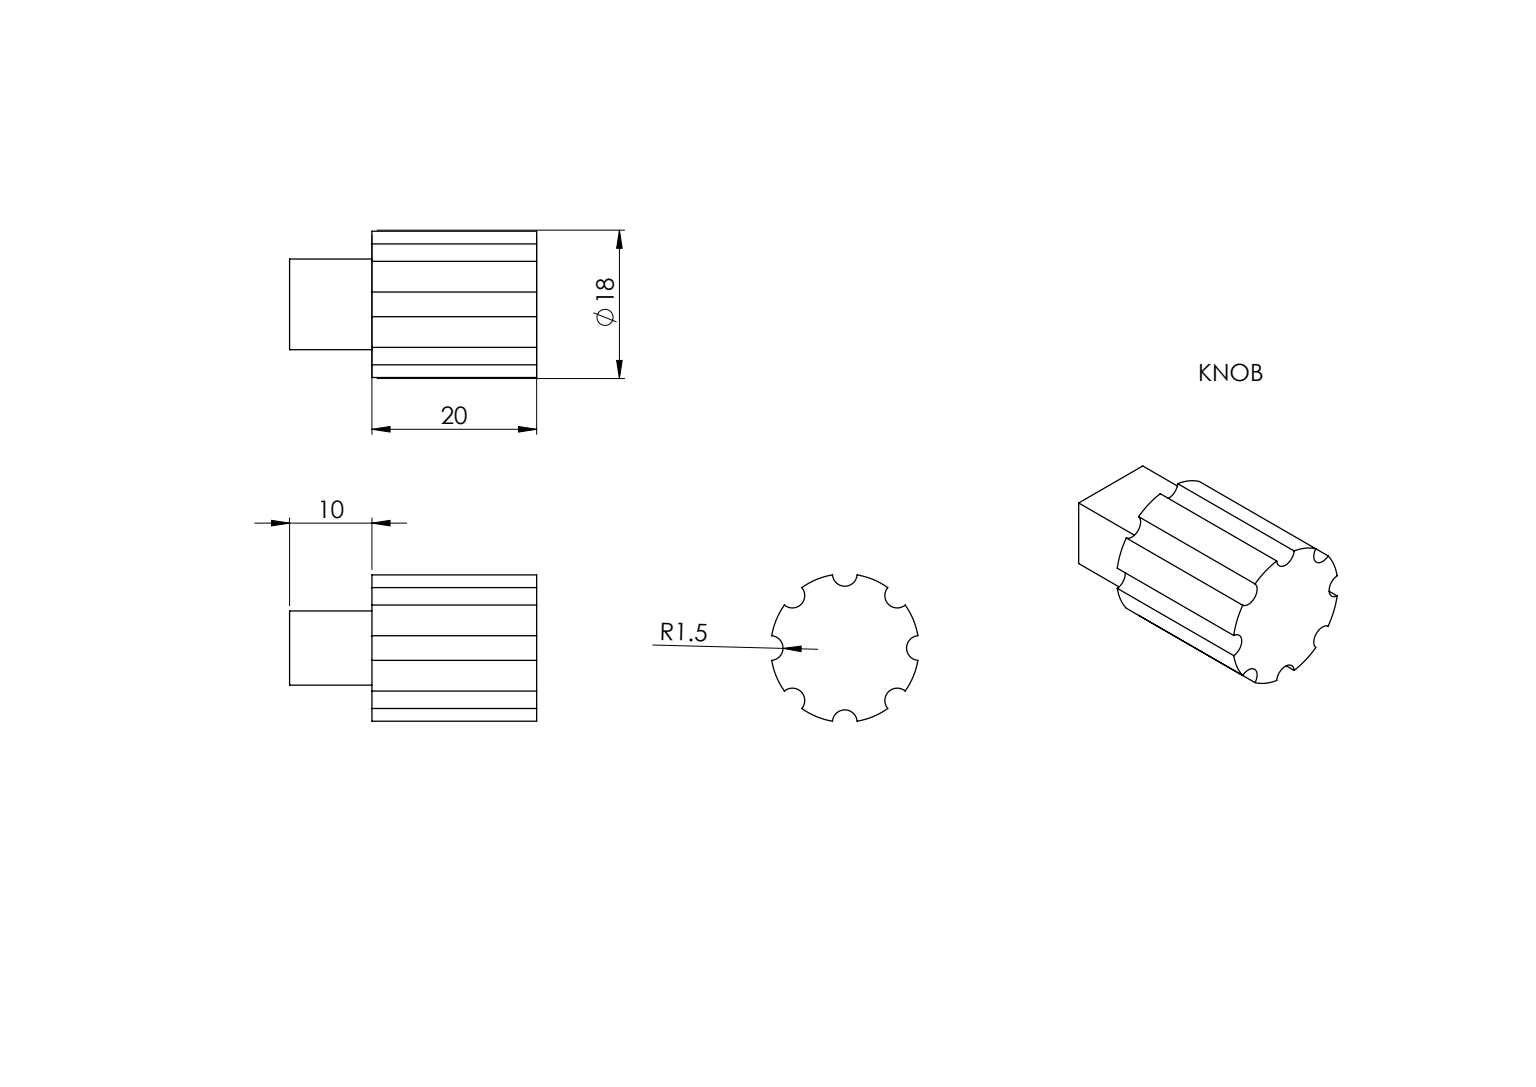
ISO-10303-21;
HEADER;
FILE_DESCRIPTION (('STEP AP214'),
    '1' );
FILE_NAME ('knob.step',
    '2026-10-26T05:42:23',
    ( '' ),
    ( '' ),
    'SwSTEP 2.0',
    'SolidWorks 2026',
    '' );
FILE_SCHEMA (( 'AUTOMOTIVE_DESIGN' ));
ENDSEC;

DATA;
#46=PLANE ( 'NONE',  #66233 ) ;
#122=DIRECTION ( 'NONE',  ( 0.000000000000000000, 0.000000000000000000, -1.000000000000000000 ) ) ;
#188=ORIENTED_EDGE ( 'NONE', *, *, #4935, .T. ) ;
#431=EDGE_CURVE ( 'NONE', #55385, #17600, #60203, .T. ) ;
#446=EDGE_CURVE ( 'NONE', #17600, #24863, #53958, .T. ) ;
#519=EDGE_LOOP ( 'NONE', ( #17956, #34557, #55612, #8707 ) ) ;
#549=DIRECTION ( 'NONE',  ( 0.000000000000000000, 1.000000000000000000, -6.195440985631455317E-17 ) ) ;
#573=EDGE_LOOP ( 'NONE', ( #31473, #72505, #31464, #35325 ) ) ;
#620=AXIS2_PLACEMENT_3D ( 'NONE', #43170, #25435, #32078 ) ;
#671=AXIS2_PLACEMENT_3D ( 'NONE', #60394, #71870, #49704 ) ;
#754=AXIS2_PLACEMENT_3D ( 'NONE', #48020, #47643, #36558 ) ;
#808=DIRECTION ( 'NONE',  ( 0.000000000000000000, 1.000000000000000000, -8.673617379884036705E-17 ) ) ;
#1050=CARTESIAN_POINT ( 'NONE',  ( 65.00000000000000000, 9.000000000000000000, 0.000000000000000000 ) ) ;
#1080=ADVANCED_FACE ( 'NONE', ( #48229 ), #31963, .F. ) ;
#1197=EDGE_CURVE ( 'NONE', #48448, #47360, #14965, .T. ) ;
#1199=DIRECTION ( 'NONE',  ( 0.000000000000000000, 0.000000000000000000, 1.000000000000000000 ) ) ;
#1357=LINE ( 'NONE', #23866, #61936 ) ;
#1404=DIRECTION ( 'NONE',  ( 1.000000000000000000, 0.000000000000000000, 0.000000000000000000 ) ) ;
#1445=DIRECTION ( 'NONE',  ( 1.000000000000000000, 0.000000000000000000, 0.000000000000000000 ) ) ;
#1478=ADVANCED_FACE ( 'NONE', ( #27429 ), #9339, .F. ) ;
#1544=ORIENTED_EDGE ( 'NONE', *, *, #61840, .F. ) ;
#1549=DIRECTION ( 'NONE',  ( 0.000000000000000000, 0.000000000000000000, -1.000000000000000000 ) ) ;
#1681=CARTESIAN_POINT ( 'NONE',  ( 45.00000000000000000, 4.500000000000001776, 5.500000000000000000 ) ) ;
#1739=ORIENTED_EDGE ( 'NONE', *, *, #12260, .F. ) ;
#1799=CARTESIAN_POINT ( 'NONE',  ( 50.00000000000000000, -5.218601775200160553, -7.332543590861066107 ) ) ;
#1839=CARTESIAN_POINT ( 'NONE',  ( 65.00000000000000000, 0.000000000000000000, 0.000000000000000000 ) ) ;
#1840=CARTESIAN_POINT ( 'NONE',  ( 45.00000000000000000, 5.218601775200101045, -7.332543590861111404 ) ) ;
#1886=UNCERTAINTY_MEASURE_WITH_UNIT (LENGTH_MEASURE( 1.000000000000000082E-05 ), #37411, 'distance_accuracy_value', 'NONE');
#1997=VECTOR ( 'NONE', #2916, 1000.000000000000000 ) ;
#2011=DIRECTION ( 'NONE',  ( 0.000000000000000000, 0.000000000000000000, 1.000000000000000000 ) ) ;
#2338=EDGE_CURVE ( 'NONE', #68777, #36937, #65592, .T. ) ;
#2553=CARTESIAN_POINT ( 'NONE',  ( 50.00000000000000000, -5.218601775200058412, 7.332543590861138938 ) ) ;
#2641=VERTEX_POINT ( 'NONE', #50445 ) ;
#2674=EDGE_CURVE ( 'NONE', #33629, #44223, #22352, .T. ) ;
#2860=VECTOR ( 'NONE', #1404, 1000.000000000000000 ) ;
#2916=DIRECTION ( 'NONE',  ( 1.000000000000000000, -0.000000000000000000, -0.000000000000000000 ) ) ;
#3084=DIRECTION ( 'NONE',  ( 0.000000000000000000, 0.000000000000000000, -1.000000000000000000 ) ) ;
#3091=CARTESIAN_POINT ( 'NONE',  ( 45.00000000000000000, 2.500000000000000444, 3.499999999999999112 ) ) ;
#3094=DIRECTION ( 'NONE',  ( 1.000000000000000000, 0.000000000000000000, 0.000000000000000000 ) ) ;
#3140=EDGE_CURVE ( 'NONE', #72600, #46789, #39515, .T. ) ;
#3192=DIRECTION ( 'NONE',  ( 1.000000000000000000, 0.000000000000000000, 0.000000000000000000 ) ) ;
#3258=LINE ( 'NONE', #42776, #39487 ) ;
#3267=ORIENTED_EDGE ( 'NONE', *, *, #14679, .F. ) ;
#3334=EDGE_CURVE ( 'NONE', #68472, #39806, #37194, .T. ) ;
#3337=ORIENTED_EDGE ( 'NONE', *, *, #39334, .T. ) ;
#3340=UNCERTAINTY_MEASURE_WITH_UNIT (LENGTH_MEASURE( 1.000000000000000082E-05 ), #12739, 'distance_accuracy_value', 'NONE');
#3447=EDGE_CURVE ( 'NONE', #60259, #55385, #31156, .T. ) ;
#3560=CYLINDRICAL_SURFACE ( 'NONE', #58366, 9.000000000000000000 ) ;
#3827=ORIENTED_EDGE ( 'NONE', *, *, #69060, .T. ) ;
#3861=( NAMED_UNIT ( * ) PLANE_ANGLE_UNIT ( ) SI_UNIT ( $, .RADIAN. ) );
#3977=ADVANCED_FACE ( 'NONE', ( #20799 ), #51796, .T. ) ;
#4098=VECTOR ( 'NONE', #808, 1000.000000000000000 ) ;
#4198=ORIENTED_EDGE ( 'NONE', *, *, #50924, .F. ) ;
#4229=LINE ( 'NONE', #20454, #24997 ) ;
#4245=CARTESIAN_POINT ( 'NONE',  ( 45.00000000000000000, -8.874999999999998224, -1.494782592887687667 ) ) ;
#4388=CIRCLE ( 'NONE', #39822, 1.500000000000000444 ) ;
#4552=CYLINDRICAL_SURFACE ( 'NONE', #62031, 9.000000000000000000 ) ;
#4729=EDGE_LOOP ( 'NONE', ( #3827, #37731, #11039, #19045 ) ) ;
#4935=EDGE_CURVE ( 'NONE', #51755, #8633, #30167, .T. ) ;
#4977=APPLICATION_CONTEXT ( 'automotive_design' ) ;
#5076=DIRECTION ( 'NONE',  ( 0.000000000000000000, -1.000000000000000000, 8.673617379884035472E-17 ) ) ;
#5100=FACE_OUTER_BOUND ( 'NONE', #43855, .T. ) ;
#5207=DIRECTION ( 'NONE',  ( 0.000000000000000000, 0.000000000000000000, 1.000000000000000000 ) ) ;
#5299=DIRECTION ( 'NONE',  ( 1.000000000000000000, 0.000000000000000000, 0.000000000000000000 ) ) ;
#5322=EDGE_LOOP ( 'NONE', ( #46801, #7370, #39720, #23204 ) ) ;
#5374=CARTESIAN_POINT ( 'NONE',  ( 34.99999999999999289, 4.500000000000000888, -3.500000000000000000 ) ) ;
#5407=DIRECTION ( 'NONE',  ( 1.000000000000000000, 0.000000000000000000, 0.000000000000000000 ) ) ;
#5416=CIRCLE ( 'NONE', #33712, 1.500000000000000444 ) ;
#5432=CARTESIAN_POINT ( 'NONE',  ( 45.00000000000000000, 8.874999999999998224, -1.494782592887687667 ) ) ;
#5621=DIRECTION ( 'NONE',  ( 0.000000000000000000, 0.000000000000000000, -1.000000000000000000 ) ) ;
#5634=ORIENTED_EDGE ( 'NONE', *, *, #39334, .F. ) ;
#5721=FACE_OUTER_BOUND ( 'NONE', #31390, .T. ) ;
#5792=DIRECTION ( 'NONE',  ( 0.000000000000000000, 0.000000000000000000, -1.000000000000000000 ) ) ;
#5818=DIRECTION ( 'NONE',  ( 1.000000000000000000, 0.000000000000000000, 0.000000000000000000 ) ) ;
#6009=ORIENTED_EDGE ( 'NONE', *, *, #59897, .T. ) ;
#6065=LINE ( 'NONE', #50774, #72936 ) ;
#6162=CARTESIAN_POINT ( 'NONE',  ( 20.78732959644809952, -4.500000000000000000, 3.499999999999999556 ) ) ;
#6210=LINE ( 'NONE', #29469, #72836 ) ;
#6340=CARTESIAN_POINT ( 'NONE',  ( 65.00000000000000000, 0.000000000000000000, 0.000000000000000000 ) ) ;
#6410=CARTESIAN_POINT ( 'NONE',  ( 20.78732959644809952, 2.500000000000000000, -3.500000000000000000 ) ) ;
#6440=CARTESIAN_POINT ( 'NONE',  ( 65.00000000000000000, 0.000000000000000000, 0.000000000000000000 ) ) ;
#6514=AXIS2_PLACEMENT_3D ( 'NONE', #1050, #6585, #34643 ) ;
#6563=CARTESIAN_POINT ( 'NONE',  ( 65.00000000000000000, 0.000000000000000000, 0.000000000000000000 ) ) ;
#6585=DIRECTION ( 'NONE',  ( 1.000000000000000000, 0.000000000000000000, 0.000000000000000000 ) ) ;
#6617=FACE_OUTER_BOUND ( 'NONE', #71782, .T. ) ;
#6766=CARTESIAN_POINT ( 'NONE',  ( 34.99999999999999289, 4.500000000000001776, 5.500000000000000000 ) ) ;
#6767=EDGE_CURVE ( 'NONE', #64526, #8633, #16230, .T. ) ;
#6789=DIRECTION ( 'NONE',  ( 1.000000000000000000, 0.000000000000000000, 0.000000000000000000 ) ) ;
#6936=LINE ( 'NONE', #29467, #2860 ) ;
#6938=DIRECTION ( 'NONE',  ( 0.000000000000000000, 0.000000000000000000, -1.000000000000000000 ) ) ;
#7332=CIRCLE ( 'NONE', #48642, 9.000000000000000000 ) ;
#7370=ORIENTED_EDGE ( 'NONE', *, *, #56475, .F. ) ;
#7405=CARTESIAN_POINT ( 'NONE',  ( 65.00000000000000000, 6.363961030679004871, 4.863961030678849440 ) ) ;
#7407=ORIENTED_EDGE ( 'NONE', *, *, #29897, .F. ) ;
#7523=DIRECTION ( 'NONE',  ( 1.000000000000000000, 0.000000000000000000, 0.000000000000000000 ) ) ;
#7603=ORIENTED_EDGE ( 'NONE', *, *, #11775, .F. ) ;
#7713=CIRCLE ( 'NONE', #28956, 9.000000000000000000 ) ;
#7806=ORIENTED_EDGE ( 'NONE', *, *, #32061, .F. ) ;
#7890=DIRECTION ( 'NONE',  ( 0.000000000000000000, 1.000000000000000000, -1.040834085586083941E-14 ) ) ;
#8017=CARTESIAN_POINT ( 'NONE',  ( 34.99999999999999289, -6.363961030678871644, 6.363961030678982667 ) ) ;
#8062=DIRECTION ( 'NONE',  ( 0.000000000000000000, -1.000000000000000000, 8.673617379884035472E-17 ) ) ;
#8100=CARTESIAN_POINT ( 'NONE',  ( 50.00000000000000000, 5.218601775200211179, 7.332543590861028804 ) ) ;
#8189=EDGE_CURVE ( 'NONE', #41205, #2641, #69341, .T. ) ;
#8354=CARTESIAN_POINT ( 'NONE',  ( 45.00000000000000000, 9.000000000000000000, 0.000000000000000000 ) ) ;
#8380=VERTEX_POINT ( 'NONE', #63425 ) ;
#8482=CYLINDRICAL_SURFACE ( 'NONE', #754, 9.000000000000000000 ) ;
#8572=ORIENTED_EDGE ( 'NONE', *, *, #34302, .F. ) ;
#8633=VERTEX_POINT ( 'NONE', #68982 ) ;
#8707=ORIENTED_EDGE ( 'NONE', *, *, #13371, .T. ) ;
#8966=EDGE_CURVE ( 'NONE', #68862, #2641, #49314, .T. ) ;
#9015=EDGE_CURVE ( 'NONE', #24863, #60259, #64072, .T. ) ;
#9059=VECTOR ( 'NONE', #16356, 1000.000000000000000 ) ;
#9220=FACE_OUTER_BOUND ( 'NONE', #11981, .T. ) ;
#9339=PLANE ( 'NONE',  #60749 ) ;
#9386=EDGE_CURVE ( 'NONE', #64526, #47560, #45612, .T. ) ;
#9492=DIRECTION ( 'NONE',  ( 0.000000000000000000, -0.7071067811865487940, -0.7071067811865464625 ) ) ;
#9558=EDGE_CURVE ( 'NONE', #54392, #54059, #19640, .T. ) ;
#9662=PRODUCT_DEFINITION_FORMATION_WITH_SPECIFIED_SOURCE ( 'ANY', '', #23145, .NOT_KNOWN. ) ;
#9854=CARTESIAN_POINT ( 'NONE',  ( 45.00000000000000000, 1.494782592887780703, 8.874999999999982236 ) ) ;
#10069=DIRECTION ( 'NONE',  ( 1.000000000000000000, 0.000000000000000000, -0.000000000000000000 ) ) ;
#10089=DIRECTION ( 'NONE',  ( 1.000000000000000000, 0.000000000000000000, 0.000000000000000000 ) ) ;
#10281=CIRCLE ( 'NONE', #68133, 9.000000000000000000 ) ;
#10315=ORIENTED_EDGE ( 'NONE', *, *, #59108, .T. ) ;
#10378=EDGE_LOOP ( 'NONE', ( #72738, #63812, #49845, #54740 ) ) ;
#10404=ORIENTED_EDGE ( 'NONE', *, *, #2674, .T. ) ;
#10489=DIRECTION ( 'NONE',  ( 0.000000000000000000, 6.195440985631455317E-17, 1.000000000000000000 ) ) ;
#10612=CARTESIAN_POINT ( 'NONE',  ( 20.78732959644809952, 2.500000000000000444, 3.499999999999999112 ) ) ;
#10639=VERTEX_POINT ( 'NONE', #53471 ) ;
#10937=LINE ( 'NONE', #43098, #24203 ) ;
#11039=ORIENTED_EDGE ( 'NONE', *, *, #18886, .F. ) ;
#11110=FACE_OUTER_BOUND ( 'NONE', #11288, .T. ) ;
#11129=ORIENTED_EDGE ( 'NONE', *, *, #67636, .T. ) ;
#11251=VECTOR ( 'NONE', #71053, 1000.000000000000000 ) ;
#11283=DIRECTION ( 'NONE',  ( 0.000000000000000000, 6.195440985631456550E-17, 1.000000000000000000 ) ) ;
#11288=EDGE_LOOP ( 'NONE', ( #69382, #49099, #26689, #56894 ) ) ;
#11325=VECTOR ( 'NONE', #66975, 1000.000000000000000 ) ;
#11376=CARTESIAN_POINT ( 'NONE',  ( 45.00000000000000000, 0.000000000000000000, 0.000000000000000000 ) ) ;
#11404=EDGE_CURVE ( 'NONE', #25148, #8380, #72157, .T. ) ;
#11461=CARTESIAN_POINT ( 'NONE',  ( 34.99999999999999289, -4.500000000000000000, -5.500000000000000000 ) ) ;
#11552=CARTESIAN_POINT ( 'NONE',  ( 65.00000000000000000, 0.000000000000000000, 0.000000000000000000 ) ) ;
#11624=VERTEX_POINT ( 'NONE', #1840 ) ;
#11775=EDGE_CURVE ( 'NONE', #25475, #39806, #52660, .T. ) ;
#11961=PRODUCT_DEFINITION_SHAPE ( 'NONE', 'NONE',  #58930 ) ;
#11981=EDGE_LOOP ( 'NONE', ( #48610, #31142, #50193, #30737 ) ) ;
#11985=CARTESIAN_POINT ( 'NONE',  ( 34.99999999999999289, -4.500000000000000000, 5.500000000000000000 ) ) ;
#12003=ORIENTED_EDGE ( 'NONE', *, *, #3447, .F. ) ;
#12064=CARTESIAN_POINT ( 'NONE',  ( 65.00000000000000000, -5.218601775200160553, -7.332543590861065219 ) ) ;
#12198=VERTEX_POINT ( 'NONE', #26552 ) ;
#12221=ORIENTED_EDGE ( 'NONE', *, *, #29224, .T. ) ;
#12260=EDGE_CURVE ( 'NONE', #8633, #25827, #53155, .T. ) ;
#12356=VECTOR ( 'NONE', #39967, 1000.000000000000000 ) ;
#12400=CIRCLE ( 'NONE', #26595, 1.500000000000000222 ) ;
#12443=AXIS2_PLACEMENT_3D ( 'NONE', #40121, #34556, #57084 ) ;
#12590=ADVANCED_FACE ( 'NONE', ( #58268 ), #18742, .T. ) ;
#12739=( LENGTH_UNIT ( ) NAMED_UNIT ( * ) SI_UNIT ( .MILLI., .METRE. ) );
#12784=DIRECTION ( 'NONE',  ( 1.000000000000000000, -0.000000000000000000, -0.000000000000000000 ) ) ;
#12890=FACE_OUTER_BOUND ( 'NONE', #72920, .T. ) ;
#13193=DIRECTION ( 'NONE',  ( 0.000000000000000000, 0.000000000000000000, -1.000000000000000000 ) ) ;
#13214=EDGE_CURVE ( 'NONE', #12198, #11624, #4388, .T. ) ;
#13314=DIRECTION ( 'NONE',  ( 0.000000000000000000, -1.000000000000000000, 8.673617379884035472E-17 ) ) ;
#13329=CYLINDRICAL_SURFACE ( 'NONE', #49034, 1.500000000000000444 ) ;
#13371=EDGE_CURVE ( 'NONE', #11624, #54715, #37815, .T. ) ;
#13381=ORIENTED_EDGE ( 'NONE', *, *, #37950, .F. ) ;
#13440=EDGE_CURVE ( 'NONE', #15065, #70677, #10281, .T. ) ;
#13450=FILL_AREA_STYLE ('',( #69271 ) ) ;
#13621=DIRECTION ( 'NONE',  ( 1.000000000000000000, 0.000000000000000000, 0.000000000000000000 ) ) ;
#13772=DIRECTION ( 'NONE',  ( 0.000000000000000000, -0.7071067811865437980, 0.7071067811865512365 ) ) ;
#13869=DIRECTION ( 'NONE',  ( 1.000000000000000000, 0.000000000000000000, 0.000000000000000000 ) ) ;
#13928=CARTESIAN_POINT ( 'NONE',  ( 65.00000000000000000, 0.000000000000000000, 0.000000000000000000 ) ) ;
#14163=DIRECTION ( 'NONE',  ( 1.000000000000000000, 0.000000000000000000, 0.000000000000000000 ) ) ;
#14201=EDGE_LOOP ( 'NONE', ( #69016, #43451, #47137, #36436 ) ) ;
#14235=ORIENTED_EDGE ( 'NONE', *, *, #60001, .F. ) ;
#14420=EDGE_CURVE ( 'NONE', #38626, #51755, #37426, .T. ) ;
#14618=DIRECTION ( 'NONE',  ( 1.000000000000000000, 0.000000000000000000, 0.000000000000000000 ) ) ;
#14679=EDGE_CURVE ( 'NONE', #68777, #17600, #6210, .T. ) ;
#14680=FACE_OUTER_BOUND ( 'NONE', #55695, .T. ) ;
#14866=CIRCLE ( 'NONE', #39687, 1.500000000000000444 ) ;
#14965=LINE ( 'NONE', #41589, #26542 ) ;
#14988=DIRECTION ( 'NONE',  ( 1.000000000000000000, 0.000000000000000000, 0.000000000000000000 ) ) ;
#15065=VERTEX_POINT ( 'NONE', #22613 ) ;
#15087=CARTESIAN_POINT ( 'NONE',  ( 34.99999999999999289, 2.500000000000000444, 3.499999999999999112 ) ) ;
#15230=DIRECTION ( 'NONE',  ( 0.000000000000000000, 0.000000000000000000, -1.000000000000000000 ) ) ;
#15392=ORIENTED_EDGE ( 'NONE', *, *, #30954, .F. ) ;
#15478=DIRECTION ( 'NONE',  ( 1.000000000000000000, 0.000000000000000000, 0.000000000000000000 ) ) ;
#15536=EDGE_LOOP ( 'NONE', ( #52738, #18696, #62734, #1739 ) ) ;
#15650=PRODUCT_CONTEXT ( 'NONE', #46934, 'mechanical' ) ;
#15706=ORIENTED_EDGE ( 'NONE', *, *, #3447, .T. ) ;
#15709=DIRECTION ( 'NONE',  ( 1.000000000000000000, 0.000000000000000000, 0.000000000000000000 ) ) ;
#15756=ORIENTED_EDGE ( 'NONE', *, *, #42670, .T. ) ;
#15823=AXIS2_PLACEMENT_3D ( 'NONE', #72302, #56041, #56402 ) ;
#15868=AXIS2_PLACEMENT_3D ( 'NONE', #16774, #6789, #16412 ) ;
#16230=CIRCLE ( 'NONE', #61050, 9.000000000000000000 ) ;
#16270=LINE ( 'NONE', #26644, #26503 ) ;
#16356=DIRECTION ( 'NONE',  ( 1.000000000000000000, 0.000000000000000000, 0.000000000000000000 ) ) ;
#16412=DIRECTION ( 'NONE',  ( 0.000000000000000000, 0.000000000000000000, -1.000000000000000000 ) ) ;
#16425=PLANE ( 'NONE',  #32178 ) ;
#16733=DIRECTION ( 'NONE',  ( 1.000000000000000000, -0.000000000000000000, 0.000000000000000000 ) ) ;
#16774=CARTESIAN_POINT ( 'NONE',  ( 45.00000000000000000, 6.363961030679004871, 6.363961030678849440 ) ) ;
#16796=ORIENTED_EDGE ( 'NONE', *, *, #54938, .F. ) ;
#17052=FACE_OUTER_BOUND ( 'NONE', #573, .T. ) ;
#17374=ORIENTED_EDGE ( 'NONE', *, *, #431, .F. ) ;
#17427=AXIS2_PLACEMENT_3D ( 'NONE', #61543, #5407, #27944 ) ;
#17524=DIRECTION ( 'NONE',  ( 0.000000000000000000, 0.000000000000000000, -1.000000000000000000 ) ) ;
#17526=CARTESIAN_POINT ( 'NONE',  ( 65.00000000000000000, -7.332543590861048344, 5.218601775200187198 ) ) ;
#17531=VERTEX_POINT ( 'NONE', #58303 ) ;
#17582=CARTESIAN_POINT ( 'NONE',  ( 34.99999999999999289, 6.363961030679004871, 6.363961030678849440 ) ) ;
#17600=VERTEX_POINT ( 'NONE', #20240 ) ;
#17778=DIRECTION ( 'NONE',  ( 1.000000000000000000, -0.000000000000000000, -0.000000000000000000 ) ) ;
#17956=ORIENTED_EDGE ( 'NONE', *, *, #25821, .F. ) ;
#17981=DIRECTION ( 'NONE',  ( 1.000000000000000000, 0.000000000000000000, 0.000000000000000000 ) ) ;
#18037=CYLINDRICAL_SURFACE ( 'NONE', #65444, 1.500000000000000444 ) ;
#18058=DIRECTION ( 'NONE',  ( 1.000000000000000000, 0.000000000000000000, 0.000000000000000000 ) ) ;
#18191=DIRECTION ( 'NONE',  ( -1.000000000000000000, 0.000000000000000000, -0.000000000000000000 ) ) ;
#18286=EDGE_CURVE ( 'NONE', #25347, #55385, #33884, .T. ) ;
#18312=CARTESIAN_POINT ( 'NONE',  ( 45.00000000000000000, 0.000000000000000000, 0.000000000000000000 ) ) ;
#18357=FACE_BOUND ( 'NONE', #36376, .T. ) ;
#18431=CARTESIAN_POINT ( 'NONE',  ( 45.00000000000000000, -4.500000000000000000, -5.500000000000000000 ) ) ;
#18589=ORIENTED_EDGE ( 'NONE', *, *, #46820, .F. ) ;
#18593=AXIS2_PLACEMENT_3D ( 'NONE', #6340, #36955, #64296 ) ;
#18633=SURFACE_STYLE_FILL_AREA ( #13450 ) ;
#18696=ORIENTED_EDGE ( 'NONE', *, *, #64237, .T. ) ;
#18742=PLANE ( 'NONE',  #30308 ) ;
#18791=DIRECTION ( 'NONE',  ( 0.000000000000000000, 0.000000000000000000, -1.000000000000000000 ) ) ;
#18850=ORIENTED_EDGE ( 'NONE', *, *, #62575, .F. ) ;
#18886=EDGE_CURVE ( 'NONE', #68472, #48472, #36214, .T. ) ;
#19014=( GEOMETRIC_REPRESENTATION_CONTEXT ( 3 ) GLOBAL_UNCERTAINTY_ASSIGNED_CONTEXT ( ( #57285 ) ) GLOBAL_UNIT_ASSIGNED_CONTEXT ( ( #53357, #41912, #64802 ) ) REPRESENTATION_CONTEXT ( 'NONE', 'WORKASPACE' ) );
#19042=ORIENTED_EDGE ( 'NONE', *, *, #67227, .F. ) ;
#19045=ORIENTED_EDGE ( 'NONE', *, *, #26050, .T. ) ;
#19100=ORIENTED_EDGE ( 'NONE', *, *, #446, .T. ) ;
#19228=VERTEX_POINT ( 'NONE', #23050 ) ;
#19492=PLANE ( 'NONE',  #22949 ) ;
#19508=VECTOR ( 'NONE', #51786, 1000.000000000000000 ) ;
#19512=DIRECTION ( 'NONE',  ( 0.000000000000000000, 0.000000000000000000, -1.000000000000000000 ) ) ;
#19629=ORIENTED_EDGE ( 'NONE', *, *, #44872, .T. ) ;
#19640=CIRCLE ( 'NONE', #63305, 1.499999999999999556 ) ;
#19670=CARTESIAN_POINT ( 'NONE',  ( 45.00000000000000000, 0.000000000000000000, 0.000000000000000000 ) ) ;
#19828=FACE_OUTER_BOUND ( 'NONE', #519, .T. ) ;
#20128=DIRECTION ( 'NONE',  ( 0.000000000000000000, 0.000000000000000000, -1.000000000000000000 ) ) ;
#20153=DIRECTION ( 'NONE',  ( 0.000000000000000000, 0.000000000000000000, -1.000000000000000000 ) ) ;
#20217=DIRECTION ( 'NONE',  ( -0.000000000000000000, 8.673617379884035472E-17, 1.000000000000000000 ) ) ;
#20240=CARTESIAN_POINT ( 'NONE',  ( 45.00000000000000000, -2.499999999999999556, -3.499999999999999556 ) ) ;
#20347=ORIENTED_EDGE ( 'NONE', *, *, #45040, .T. ) ;
#20446=DIRECTION ( 'NONE',  ( 0.000000000000000000, 0.000000000000000000, -1.000000000000000000 ) ) ;
#20454=CARTESIAN_POINT ( 'NONE',  ( 34.99999999999999289, 2.500000000000000000, -3.500000000000000000 ) ) ;
#20492=CARTESIAN_POINT ( 'NONE',  ( 45.00000000000000000, -2.499999999999999556, 3.499999999999999556 ) ) ;
#20568=VECTOR ( 'NONE', #48416, 1000.000000000000000 ) ;
#20587=CARTESIAN_POINT ( 'NONE',  ( 65.00000000000000000, 0.000000000000000000, 0.000000000000000000 ) ) ;
#20611=CYLINDRICAL_SURFACE ( 'NONE', #620, 1.500000000000000444 ) ;
#20614=AXIS2_PLACEMENT_3D ( 'NONE', #11552, #39996, #1199 ) ;
#20666=EDGE_LOOP ( 'NONE', ( #33083, #22259, #69325, #19629, #7407, #33543, #69321, #28131, #50552, #68749, #28455, #3337, #39344, #24424, #24054, #38166, #51564, #1544, #56528 ) ) ;
#20714=CIRCLE ( 'NONE', #62022, 1.500000000000000666 ) ;
#20787=LINE ( 'NONE', #43344, #71482 ) ;
#20799=FACE_OUTER_BOUND ( 'NONE', #45469, .T. ) ;
#20862=AXIS2_PLACEMENT_3D ( 'NONE', #64200, #1445, #52040 ) ;
#20958=FACE_OUTER_BOUND ( 'NONE', #36572, .T. ) ;
#20993=LINE ( 'NONE', #15087, #57263 ) ;
#21022=ORIENTED_EDGE ( 'NONE', *, *, #43507, .F. ) ;
#21111=CARTESIAN_POINT ( 'NONE',  ( 65.00000000000000000, 7.332543590861157590, 5.218601775200033543 ) ) ;
#21170=ORIENTED_EDGE ( 'NONE', *, *, #46759, .T. ) ;
#21308=EDGE_CURVE ( 'NONE', #29028, #64526, #6065, .T. ) ;
#21321=LINE ( 'NONE', #66032, #44378 ) ;
#21425=FACE_OUTER_BOUND ( 'NONE', #25476, .T. ) ;
#21560=CARTESIAN_POINT ( 'NONE',  ( 65.00000000000000000, -6.363961030678871644, 6.363961030678982667 ) ) ;
#21587=EDGE_CURVE ( 'NONE', #12198, #59156, #38709, .T. ) ;
#21698=ORIENTED_EDGE ( 'NONE', *, *, #30772, .T. ) ;
#21774=VECTOR ( 'NONE', #15230, 1000.000000000000000 ) ;
#21839=AXIS2_PLACEMENT_3D ( 'NONE', #8017, #59334, #65253 ) ;
#21857=AXIS2_PLACEMENT_3D ( 'NONE', #28003, #39446, #61967 ) ;
#21974=DIRECTION ( 'NONE',  ( 1.000000000000000000, 0.000000000000000000, 0.000000000000000000 ) ) ;
#21999=MANIFOLD_SOLID_BREP ( 'CirPattern1', #47738 ) ;
#22049=CIRCLE ( 'NONE', #44487, 9.000000000000000000 ) ;
#22243=CARTESIAN_POINT ( 'NONE',  ( 50.00000000000000000, 1.494782592887768269, 8.874999999999984013 ) ) ;
#22259=ORIENTED_EDGE ( 'NONE', *, *, #25821, .T. ) ;
#22351=ORIENTED_EDGE ( 'NONE', *, *, #38259, .T. ) ;
#22352=LINE ( 'NONE', #67078, #66677 ) ;
#22381=ADVANCED_FACE ( 'NONE', ( #17052 ), #39609, .T. ) ;
#22393=CARTESIAN_POINT ( 'NONE',  ( 50.00000000000000000, -8.875000000000000000, 1.494782592887675232 ) ) ;
#22496=FACE_OUTER_BOUND ( 'NONE', #50799, .T. ) ;
#22613=CARTESIAN_POINT ( 'NONE',  ( 65.00000000000000000, 8.874999999999998224, 1.494782592887675232 ) ) ;
#22708=EDGE_CURVE ( 'NONE', #48448, #33629, #29952, .T. ) ;
#22935=ORIENTED_EDGE ( 'NONE', *, *, #46820, .T. ) ;
#22949=AXIS2_PLACEMENT_3D ( 'NONE', #53123, #36862, #8062 ) ;
#23012=VECTOR ( 'NONE', #64511, 1000.000000000000000 ) ;
#23030=ORIENTED_EDGE ( 'NONE', *, *, #13214, .T. ) ;
#23040=AXIS2_PLACEMENT_3D ( 'NONE', #45002, #72342, #34621 ) ;
#23043=CARTESIAN_POINT ( 'NONE',  ( 65.00000000000000000, -6.363961030678960462, -6.363961030678893849 ) ) ;
#23047=CIRCLE ( 'NONE', #671, 1.500000000000000222 ) ;
#23050=CARTESIAN_POINT ( 'NONE',  ( 65.00000000000000000, -1.494782592887706096, -8.874999999999992895 ) ) ;
#23072=CARTESIAN_POINT ( 'NONE',  ( 45.00000000000000000, 0.000000000000000000, 0.000000000000000000 ) ) ;
#23100=CARTESIAN_POINT ( 'NONE',  ( 0.000000000000000000, 0.000000000000000000, 0.000000000000000000 ) ) ;
#23145=PRODUCT ( 'knob', 'knob', '', ( #15650 ) ) ;
#23204=ORIENTED_EDGE ( 'NONE', *, *, #41428, .F. ) ;
#23231=VECTOR ( 'NONE', #5818, 1000.000000000000000 ) ;
#23315=CARTESIAN_POINT ( 'NONE',  ( 45.00000000000000000, 4.500000000000000888, -3.500000000000000000 ) ) ;
#23335=FACE_OUTER_BOUND ( 'NONE', #35526, .T. ) ;
#23612=CARTESIAN_POINT ( 'NONE',  ( 34.99999999999999289, -3.142333204958820020E-14, -9.000000000000000000 ) ) ;
#23694=CARTESIAN_POINT ( 'NONE',  ( 34.99999999999999289, 6.363961030679004871, 4.863961030678849440 ) ) ;
#23746=LINE ( 'NONE', #46294, #28538 ) ;
#23765=AXIS2_PLACEMENT_3D ( 'NONE', #23100, #68190, #46012 ) ;
#23780=CARTESIAN_POINT ( 'NONE',  ( 65.00000000000000000, 1.494782592887643924, -8.875000000000003553 ) ) ;
#23866=CARTESIAN_POINT ( 'NONE',  ( 50.00000000000000000, 8.875000000000000000, -1.494782592887675232 ) ) ;
#24025=PRODUCT_DEFINITION_CONTEXT ( 'detailed design', #4977, 'design' ) ;
#24054=ORIENTED_EDGE ( 'NONE', *, *, #11775, .T. ) ;
#24187=DIRECTION ( 'NONE',  ( 0.000000000000000000, 6.195440985631455317E-17, 1.000000000000000000 ) ) ;
#24203=VECTOR ( 'NONE', #27208, 1000.000000000000000 ) ;
#24424=ORIENTED_EDGE ( 'NONE', *, *, #33157, .F. ) ;
#24452=ORIENTED_EDGE ( 'NONE', *, *, #29897, .T. ) ;
#24480=ORIENTED_EDGE ( 'NONE', *, *, #58454, .T. ) ;
#24739=ORIENTED_EDGE ( 'NONE', *, *, #9015, .F. ) ;
#24799=ORIENTED_EDGE ( 'NONE', *, *, #30402, .T. ) ;
#24863=VERTEX_POINT ( 'NONE', #27180 ) ;
#24882=CARTESIAN_POINT ( 'NONE',  ( 65.00000000000000000, -5.218601775200058412, 7.332543590861138050 ) ) ;
#24918=ORIENTED_EDGE ( 'NONE', *, *, #34570, .T. ) ;
#24944=EDGE_CURVE ( 'NONE', #10639, #56113, #51287, .T. ) ;
#24997=VECTOR ( 'NONE', #10489, 1000.000000000000000 ) ;
#25132=CARTESIAN_POINT ( 'NONE',  ( 34.99999999999999289, 2.500000000000000444, 5.500000000000000000 ) ) ;
#25148=VERTEX_POINT ( 'NONE', #33077 ) ;
#25212=CARTESIAN_POINT ( 'NONE',  ( 34.99999999999999289, -2.499999999999999556, 3.499999999999999556 ) ) ;
#25255=EDGE_CURVE ( 'NONE', #25148, #48448, #55980, .T. ) ;
#25347=VERTEX_POINT ( 'NONE', #64043 ) ;
#25435=DIRECTION ( 'NONE',  ( 1.000000000000000000, -0.000000000000000000, -0.000000000000000000 ) ) ;
#25475=VERTEX_POINT ( 'NONE', #17526 ) ;
#25476=EDGE_LOOP ( 'NONE', ( #56251, #14235, #24452, #25615 ) ) ;
#25507=CARTESIAN_POINT ( 'NONE',  ( 45.00000000000000000, 6.363961030679004871, 4.863961030678849440 ) ) ;
#25615=ORIENTED_EDGE ( 'NONE', *, *, #38259, .F. ) ;
#25619=ORIENTED_EDGE ( 'NONE', *, *, #9386, .F. ) ;
#25657=CARTESIAN_POINT ( 'NONE',  ( 45.00000000000000000, 2.500000000000000000, -3.500000000000000000 ) ) ;
#25821=EDGE_CURVE ( 'NONE', #33507, #54715, #30021, .T. ) ;
#25827=VERTEX_POINT ( 'NONE', #24882 ) ;
#26030=CARTESIAN_POINT ( 'NONE',  ( 34.99999999999999289, 9.426999614876460059E-14, 7.499999999999999112 ) ) ;
#26050=EDGE_CURVE ( 'NONE', #68472, #66931, #16270, .T. ) ;
#26142=CARTESIAN_POINT ( 'NONE',  ( 65.00000000000000000, -3.142333204958820020E-14, -9.000000000000000000 ) ) ;
#26412=CARTESIAN_POINT ( 'NONE',  ( 65.00000000000000000, 6.363961030679004871, 6.363961030678849440 ) ) ;
#26499=VECTOR ( 'NONE', #65390, 1000.000000000000000 ) ;
#26503=VECTOR ( 'NONE', #37711, 1000.000000000000000 ) ;
#26534=CIRCLE ( 'NONE', #45370, 1.500000000000000222 ) ;
#26539=FACE_OUTER_BOUND ( 'NONE', #28983, .T. ) ;
#26542=VECTOR ( 'NONE', #13869, 1000.000000000000000 ) ;
#26552=CARTESIAN_POINT ( 'NONE',  ( 45.00000000000000000, 7.332543590861092753, -5.218601775200125914 ) ) ;
#26595=AXIS2_PLACEMENT_3D ( 'NONE', #21560, #48922, #44114 ) ;
#26602=CIRCLE ( 'NONE', #65506, 9.000000000000000000 ) ;
#26608=CIRCLE ( 'NONE', #43165, 1.500000000000000444 ) ;
#26644=CARTESIAN_POINT ( 'NONE',  ( 50.00000000000000000, -8.875000000000000000, -1.494782592887675232 ) ) ;
#26689=ORIENTED_EDGE ( 'NONE', *, *, #35579, .F. ) ;
#26720=DIRECTION ( 'NONE',  ( 0.000000000000000000, 1.000000000000000000, -6.195440985631456550E-17 ) ) ;
#26881=LINE ( 'NONE', #42405, #72473 ) ;
#26896=VECTOR ( 'NONE', #24187, 1000.000000000000000 ) ;
#27067=( NAMED_UNIT ( * ) SI_UNIT ( $, .STERADIAN. ) SOLID_ANGLE_UNIT ( ) );
#27081=DIRECTION ( 'NONE',  ( -1.000000000000000000, -0.000000000000000000, -0.000000000000000000 ) ) ;
#27152=CARTESIAN_POINT ( 'NONE',  ( 45.00000000000000000, 2.500000000000000444, 3.499999999999999112 ) ) ;
#27180=CARTESIAN_POINT ( 'NONE',  ( 45.00000000000000000, 2.500000000000000000, -3.500000000000000000 ) ) ;
#27208=DIRECTION ( 'NONE',  ( 1.000000000000000000, -0.000000000000000000, -0.000000000000000000 ) ) ;
#27330=ADVANCED_FACE ( 'NONE', ( #21425 ), #27715, .F. ) ;
#27429=FACE_OUTER_BOUND ( 'NONE', #36560, .T. ) ;
#27437=AXIS2_PLACEMENT_3D ( 'NONE', #43454, #48625, #59690 ) ;
#27715=CYLINDRICAL_SURFACE ( 'NONE', #35968, 1.500000000000000444 ) ;
#27818=ORIENTED_EDGE ( 'NONE', *, *, #49856, .F. ) ;
#27821=ADVANCED_FACE ( 'NONE', ( #26539 ), #20611, .F. ) ;
#27870=DIRECTION ( 'NONE',  ( 0.000000000000000000, 0.000000000000000000, -1.000000000000000000 ) ) ;
#27944=DIRECTION ( 'NONE',  ( 0.000000000000000000, 0.000000000000000000, -1.000000000000000000 ) ) ;
#28003=CARTESIAN_POINT ( 'NONE',  ( 45.00000000000000000, 0.000000000000000000, 0.000000000000000000 ) ) ;
#28008=AXIS2_PLACEMENT_3D ( 'NONE', #52725, #69368, #6938 ) ;
#28064=CARTESIAN_POINT ( 'NONE',  ( 34.99999999999999289, -9.000000000000000000, 0.000000000000000000 ) ) ;
#28104=ORIENTED_EDGE ( 'NONE', *, *, #69060, .F. ) ;
#28131=ORIENTED_EDGE ( 'NONE', *, *, #59897, .F. ) ;
#28309=ADVANCED_FACE ( 'NONE', ( #5100, #44990 ), #67528, .F. ) ;
#28331=PLANE ( 'NONE',  #31300 ) ;
#28455=ORIENTED_EDGE ( 'NONE', *, *, #33822, .F. ) ;
#28489=MECHANICAL_DESIGN_GEOMETRIC_PRESENTATION_REPRESENTATION('',(#39139),#63903);
#28538=VECTOR ( 'NONE', #18191, 1000.000000000000000 ) ;
#28694=CARTESIAN_POINT ( 'NONE',  ( 50.00000000000000000, 7.332543590861156702, 5.218601775200032655 ) ) ;
#28773=DIRECTION ( 'NONE',  ( 1.000000000000000000, -0.000000000000000000, -0.000000000000000000 ) ) ;
#28872=ADVANCED_FACE ( 'NONE', ( #36068 ), #3560, .T. ) ;
#28956=AXIS2_PLACEMENT_3D ( 'NONE', #1839, #13621, #18791 ) ;
#28964=AXIS2_PLACEMENT_3D ( 'NONE', #37805, #55175, #71431 ) ;
#28983=EDGE_LOOP ( 'NONE', ( #21022, #62018, #18850, #6009 ) ) ;
#29028=VERTEX_POINT ( 'NONE', #53058 ) ;
#29071=ADVANCED_FACE ( 'NONE', ( #59686 ), #31255, .F. ) ;
#29122=AXIS2_PLACEMENT_3D ( 'NONE', #20587, #43513, #66404 ) ;
#29224=EDGE_CURVE ( 'NONE', #36937, #24863, #56652, .T. ) ;
#29467=CARTESIAN_POINT ( 'NONE',  ( 20.78732959644809952, -4.500000000000000000, -5.500000000000000000 ) ) ;
#29469=CARTESIAN_POINT ( 'NONE',  ( 20.78732959644809952, -2.499999999999999556, -3.499999999999999556 ) ) ;
#29591=LINE ( 'NONE', #34764, #4098 ) ;
#29897=EDGE_CURVE ( 'NONE', #15065, #57451, #64284, .T. ) ;
#29901=ORIENTED_EDGE ( 'NONE', *, *, #37581, .T. ) ;
#29952=LINE ( 'NONE', #25132, #53391 ) ;
#29982=VERTEX_POINT ( 'NONE', #52369 ) ;
#30021=CIRCLE ( 'NONE', #71312, 9.000000000000000000 ) ;
#30104=CARTESIAN_POINT ( 'NONE',  ( 45.00000000000000000, 9.426999614876460059E-14, 7.499999999999999112 ) ) ;
#30167=CIRCLE ( 'NONE', #47847, 1.500000000000000444 ) ;
#30249=AXIS2_PLACEMENT_3D ( 'NONE', #66100, #15478, #65364 ) ;
#30308=AXIS2_PLACEMENT_3D ( 'NONE', #47565, #30932, #53473 ) ;
#30386=CARTESIAN_POINT ( 'NONE',  ( 65.00000000000000000, -7.332543590861121174, -5.218601775200084170 ) ) ;
#30402=EDGE_CURVE ( 'NONE', #71147, #39806, #61916, .T. ) ;
#30465=SURFACE_SIDE_STYLE ('',( #18633 ) ) ;
#30538=CARTESIAN_POINT ( 'NONE',  ( 50.00000000000000000, -7.332543590861121174, -5.218601775200084170 ) ) ;
#30563=CARTESIAN_POINT ( 'NONE',  ( 45.00000000000000000, 0.000000000000000000, 0.000000000000000000 ) ) ;
#30710=ORIENTED_EDGE ( 'NONE', *, *, #57824, .F. ) ;
#30737=ORIENTED_EDGE ( 'NONE', *, *, #56475, .T. ) ;
#30772=EDGE_CURVE ( 'NONE', #17531, #56113, #31332, .T. ) ;
#30874=ORIENTED_EDGE ( 'NONE', *, *, #13440, .F. ) ;
#30883=CARTESIAN_POINT ( 'NONE',  ( 65.00000000000000000, 0.000000000000000000, 0.000000000000000000 ) ) ;
#30886=DIRECTION ( 'NONE',  ( 0.000000000000000000, 0.000000000000000000, 1.000000000000000000 ) ) ;
#30932=DIRECTION ( 'NONE',  ( 1.000000000000000000, 0.000000000000000000, 0.000000000000000000 ) ) ;
#30954=EDGE_CURVE ( 'NONE', #38626, #71147, #26602, .T. ) ;
#30956=DIRECTION ( 'NONE',  ( 0.000000000000000000, 0.000000000000000000, -1.000000000000000000 ) ) ;
#31142=ORIENTED_EDGE ( 'NONE', *, *, #34302, .T. ) ;
#31149=PLANE ( 'NONE',  #61989 ) ;
#31156=LINE ( 'NONE', #3091, #11251 ) ;
#31255=PLANE ( 'NONE',  #34820 ) ;
#31289=AXIS2_PLACEMENT_3D ( 'NONE', #23072, #50800, #17524 ) ;
#31299=ORIENTED_EDGE ( 'NONE', *, *, #44872, .F. ) ;
#31300=AXIS2_PLACEMENT_3D ( 'NONE', #6162, #45328, #67864 ) ;
#31332=CIRCLE ( 'NONE', #28964, 1.500000000000000444 ) ;
#31390=EDGE_LOOP ( 'NONE', ( #54504, #12221, #54418, #45493 ) ) ;
#31464=ORIENTED_EDGE ( 'NONE', *, *, #24944, .F. ) ;
#31473=ORIENTED_EDGE ( 'NONE', *, *, #3140, .T. ) ;
#31534=CARTESIAN_POINT ( 'NONE',  ( 65.00000000000000000, 0.000000000000000000, 0.000000000000000000 ) ) ;
#31569=ORIENTED_EDGE ( 'NONE', *, *, #42670, .F. ) ;
#31692=CYLINDRICAL_SURFACE ( 'NONE', #29122, 9.000000000000000000 ) ;
#31825=CYLINDRICAL_SURFACE ( 'NONE', #46307, 1.500000000000000444 ) ;
#31836=ADVANCED_FACE ( 'NONE', ( #12890 ), #35423, .F. ) ;
#31905=DIRECTION ( 'NONE',  ( 1.000000000000000000, 0.000000000000000000, 0.000000000000000000 ) ) ;
#31963=CYLINDRICAL_SURFACE ( 'NONE', #53687, 1.500000000000000444 ) ;
#31991=CARTESIAN_POINT ( 'NONE',  ( 65.00000000000000000, 0.000000000000000000, 0.000000000000000000 ) ) ;
#32022=EDGE_CURVE ( 'NONE', #68374, #60259, #41697, .T. ) ;
#32052=DIRECTION ( 'NONE',  ( 1.000000000000000000, 0.000000000000000000, 0.000000000000000000 ) ) ;
#32057=CARTESIAN_POINT ( 'NONE',  ( 45.00000000000000000, 1.494782592887656580, -8.875000000000001776 ) ) ;
#32061=EDGE_CURVE ( 'NONE', #54392, #11624, #44332, .T. ) ;
#32078=DIRECTION ( 'NONE',  ( 0.000000000000000000, 0.000000000000000000, -1.000000000000000000 ) ) ;
#32153=EDGE_CURVE ( 'NONE', #2641, #70677, #57843, .T. ) ;
#32177=CARTESIAN_POINT ( 'NONE',  ( 45.00000000000000000, -6.363961030678871644, 6.363961030678982667 ) ) ;
#32178=AXIS2_PLACEMENT_3D ( 'NONE', #68148, #549, #38983 ) ;
#32252=CARTESIAN_POINT ( 'NONE',  ( 45.00000000000000000, -9.000000000000000000, 0.000000000000000000 ) ) ;
#32383=DIRECTION ( 'NONE',  ( -1.000000000000000000, 0.000000000000000000, 0.000000000000000000 ) ) ;
#32950=ORIENTED_EDGE ( 'NONE', *, *, #9558, .F. ) ;
#33077=CARTESIAN_POINT ( 'NONE',  ( 34.99999999999999289, 4.500000000000000888, -5.500000000000000888 ) ) ;
#33083=ORIENTED_EDGE ( 'NONE', *, *, #49669, .F. ) ;
#33157=EDGE_CURVE ( 'NONE', #25475, #40213, #23047, .T. ) ;
#33217=ORIENTED_EDGE ( 'NONE', *, *, #21308, .F. ) ;
#33358=CARTESIAN_POINT ( 'NONE',  ( 20.78732959644809952, 4.500000000000000888, -5.500000000000000888 ) ) ;
#33361=CARTESIAN_POINT ( 'NONE',  ( 45.00000000000000000, 0.000000000000000000, 0.000000000000000000 ) ) ;
#33507=VERTEX_POINT ( 'NONE', #23780 ) ;
#33543=ORIENTED_EDGE ( 'NONE', *, *, #13440, .T. ) ;
#33544=VECTOR ( 'NONE', #57194, 1000.000000000000000 ) ;
#33581=CARTESIAN_POINT ( 'NONE',  ( 34.99999999999999289, 9.426999614876460059E-14, 9.000000000000000000 ) ) ;
#33590=CIRCLE ( 'NONE', #43037, 1.500000000000000888 ) ;
#33629=VERTEX_POINT ( 'NONE', #11985 ) ;
#33639=DIRECTION ( 'NONE',  ( -1.000000000000000000, 0.000000000000000000, 0.000000000000000000 ) ) ;
#33665=VECTOR ( 'NONE', #54515, 1000.000000000000000 ) ;
#33712=AXIS2_PLACEMENT_3D ( 'NONE', #47055, #7523, #7890 ) ;
#33822=EDGE_CURVE ( 'NONE', #29028, #17531, #5416, .T. ) ;
#33884=LINE ( 'NONE', #60868, #23231 ) ;
#33931=DIRECTION ( 'NONE',  ( 1.000000000000000000, 0.000000000000000000, 0.000000000000000000 ) ) ;
#34302=EDGE_CURVE ( 'NONE', #54059, #19228, #20787, .T. ) ;
#34310=CARTESIAN_POINT ( 'NONE',  ( 34.99999999999999289, 2.500000000000000000, -3.500000000000000000 ) ) ;
#34487=ADVANCED_FACE ( 'NONE', ( #55154 ), #4552, .T. ) ;
#34556=DIRECTION ( 'NONE',  ( 1.000000000000000000, 0.000000000000000000, 0.000000000000000000 ) ) ;
#34557=ORIENTED_EDGE ( 'NONE', *, *, #37950, .T. ) ;
#34570=EDGE_CURVE ( 'NONE', #47360, #29982, #39624, .T. ) ;
#34621=DIRECTION ( 'NONE',  ( 0.000000000000000000, 1.000000000000000000, -8.673617379884036705E-17 ) ) ;
#34643=DIRECTION ( 'NONE',  ( 0.000000000000000000, 0.000000000000000000, -1.000000000000000000 ) ) ;
#34764=CARTESIAN_POINT ( 'NONE',  ( 34.99999999999999289, -2.499999999999999556, -5.500000000000000000 ) ) ;
#34786=ORIENTED_EDGE ( 'NONE', *, *, #57824, .T. ) ;
#34820=AXIS2_PLACEMENT_3D ( 'NONE', #53797, #3192, #65603 ) ;
#34877=EDGE_LOOP ( 'NONE', ( #12003, #24739, #44270, #17374 ) ) ;
#35138=ADVANCED_FACE ( 'NONE', ( #67325 ), #66582, .F. ) ;
#35325=ORIENTED_EDGE ( 'NONE', *, *, #62575, .T. ) ;
#35423=CYLINDRICAL_SURFACE ( 'NONE', #66752, 1.499999999999999556 ) ;
#35526=EDGE_LOOP ( 'NONE', ( #67566, #25619, #33217, #67516 ) ) ;
#35579=EDGE_CURVE ( 'NONE', #44223, #25148, #29591, .T. ) ;
#35731=DIRECTION ( 'NONE',  ( 0.000000000000000000, 0.000000000000000000, 1.000000000000000000 ) ) ;
#35732=EDGE_CURVE ( 'NONE', #8380, #47360, #56931, .T. ) ;
#35848=CIRCLE ( 'NONE', #15823, 1.500000000000000888 ) ;
#35968=AXIS2_PLACEMENT_3D ( 'NONE', #44714, #66881, #67250 ) ;
#36043=ORIENTED_EDGE ( 'NONE', *, *, #21308, .T. ) ;
#36068=FACE_OUTER_BOUND ( 'NONE', #54143, .T. ) ;
#36075=LINE ( 'NONE', #30538, #23012 ) ;
#36110=ORIENTED_EDGE ( 'NONE', *, *, #66718, .T. ) ;
#36214=CIRCLE ( 'NONE', #20862, 9.000000000000000000 ) ;
#36376=EDGE_LOOP ( 'NONE', ( #58926, #20347, #37529, #64912 ) ) ;
#36400=DIRECTION ( 'NONE',  ( 1.000000000000000000, 0.000000000000000000, 0.000000000000000000 ) ) ;
#36436=ORIENTED_EDGE ( 'NONE', *, *, #35732, .F. ) ;
#36558=DIRECTION ( 'NONE',  ( 0.000000000000000000, 0.000000000000000000, 1.000000000000000000 ) ) ;
#36560=EDGE_LOOP ( 'NONE', ( #41796, #65819, #19100, #41236 ) ) ;
#36572=EDGE_LOOP ( 'NONE', ( #57851, #67697, #30874, #57160 ) ) ;
#36690=DIRECTION ( 'NONE',  ( 0.000000000000000000, 6.195440985631456550E-17, 1.000000000000000000 ) ) ;
#36814=CARTESIAN_POINT ( 'NONE',  ( 34.99999999999999289, -2.499999999999999556, -3.499999999999999556 ) ) ;
#36823=CARTESIAN_POINT ( 'NONE',  ( 45.00000000000000000, 5.218601775200201409, 7.332543590861037686 ) ) ;
#36830=CARTESIAN_POINT ( 'NONE',  ( 50.00000000000000000, -7.332543590861048344, 5.218601775200186310 ) ) ;
#36862=DIRECTION ( 'NONE',  ( -0.000000000000000000, 8.673617379884035472E-17, 1.000000000000000000 ) ) ;
#36937=VERTEX_POINT ( 'NONE', #34310 ) ;
#36955=DIRECTION ( 'NONE',  ( -1.000000000000000000, -0.000000000000000000, -0.000000000000000000 ) ) ;
#37120=DIRECTION ( 'NONE',  ( 0.000000000000000000, 0.7071067811865388020, -0.7071067811865562325 ) ) ;
#37164=FACE_OUTER_BOUND ( 'NONE', #38980, .T. ) ;
#37194=CIRCLE ( 'NONE', #46627, 1.500000000000000444 ) ;
#37411=( LENGTH_UNIT ( ) NAMED_UNIT ( * ) SI_UNIT ( .MILLI., .METRE. ) );
#37426=CIRCLE ( 'NONE', #28008, 1.500000000000000444 ) ;
#37489=AXIS2_PLACEMENT_3D ( 'NONE', #11376, #17981, #61974 ) ;
#37529=ORIENTED_EDGE ( 'NONE', *, *, #61088, .T. ) ;
#37578=ADVANCED_FACE ( 'NONE', ( #53867 ), #19492, .T. ) ;
#37581=EDGE_CURVE ( 'NONE', #29982, #44755, #3258, .T. ) ;
#37711=DIRECTION ( 'NONE',  ( -1.000000000000000000, 0.000000000000000000, 0.000000000000000000 ) ) ;
#37731=ORIENTED_EDGE ( 'NONE', *, *, #41428, .T. ) ;
#37805=CARTESIAN_POINT ( 'NONE',  ( 65.00000000000000000, 9.426999614876460059E-14, 9.000000000000000000 ) ) ;
#37815=LINE ( 'NONE', #45910, #56317 ) ;
#37950=EDGE_CURVE ( 'NONE', #33507, #54392, #50150, .T. ) ;
#38148=ADVANCED_FACE ( 'NONE', ( #51598 ), #28331, .T. ) ;
#38166=ORIENTED_EDGE ( 'NONE', *, *, #3334, .F. ) ;
#38259=EDGE_CURVE ( 'NONE', #59156, #57451, #1357, .T. ) ;
#38339=VECTOR ( 'NONE', #70525, 1000.000000000000000 ) ;
#38420=CARTESIAN_POINT ( 'NONE',  ( 45.00000000000000000, 0.000000000000000000, 0.000000000000000000 ) ) ;
#38462=CARTESIAN_POINT ( 'NONE',  ( 34.99999999999999289, 0.000000000000000000, 0.000000000000000000 ) ) ;
#38526=CARTESIAN_POINT ( 'NONE',  ( 65.00000000000000000, 0.000000000000000000, 0.000000000000000000 ) ) ;
#38626=VERTEX_POINT ( 'NONE', #53035 ) ;
#38709=CIRCLE ( 'NONE', #54047, 9.000000000000000000 ) ;
#38980=EDGE_LOOP ( 'NONE', ( #58263, #44443, #71366, #3267 ) ) ;
#38983=DIRECTION ( 'NONE',  ( 0.000000000000000000, 6.195440985631455317E-17, 1.000000000000000000 ) ) ;
#39072=ORIENTED_EDGE ( 'NONE', *, *, #3334, .T. ) ;
#39139=STYLED_ITEM ( 'NONE', ( #64437 ), #54116 ) ;
#39334=EDGE_CURVE ( 'NONE', #29028, #25827, #44293, .T. ) ;
#39344=ORIENTED_EDGE ( 'NONE', *, *, #65317, .F. ) ;
#39366=ORIENTED_EDGE ( 'NONE', *, *, #67227, .T. ) ;
#39428=DIRECTION ( 'NONE',  ( 0.000000000000000000, 0.000000000000000000, -1.000000000000000000 ) ) ;
#39446=DIRECTION ( 'NONE',  ( 1.000000000000000000, 0.000000000000000000, 0.000000000000000000 ) ) ;
#39465=VERTEX_POINT ( 'NONE', #56370 ) ;
#39487=VECTOR ( 'NONE', #30956, 1000.000000000000000 ) ;
#39515=CIRCLE ( 'NONE', #31289, 9.000000000000000000 ) ;
#39520=VECTOR ( 'NONE', #51480, 1000.000000000000000 ) ;
#39609=CYLINDRICAL_SURFACE ( 'NONE', #18593, 9.000000000000000000 ) ;
#39624=LINE ( 'NONE', #51061, #11325 ) ;
#39655=DIRECTION ( 'NONE',  ( 0.000000000000000000, 0.000000000000000000, -1.000000000000000000 ) ) ;
#39687=AXIS2_PLACEMENT_3D ( 'NONE', #26142, #66774, #49413 ) ;
#39699=DIRECTION ( 'NONE',  ( -1.000000000000000000, 0.000000000000000000, 0.000000000000000000 ) ) ;
#39720=ORIENTED_EDGE ( 'NONE', *, *, #61840, .T. ) ;
#39728=CARTESIAN_POINT ( 'NONE',  ( 65.00000000000000000, 0.000000000000000000, 0.000000000000000000 ) ) ;
#39806=VERTEX_POINT ( 'NONE', #45652 ) ;
#39822=AXIS2_PLACEMENT_3D ( 'NONE', #55907, #5299, #20446 ) ;
#39967=DIRECTION ( 'NONE',  ( 0.000000000000000000, 6.195440985631456550E-17, 1.000000000000000000 ) ) ;
#39996=DIRECTION ( 'NONE',  ( -1.000000000000000000, -0.000000000000000000, -0.000000000000000000 ) ) ;
#40013=CARTESIAN_POINT ( 'NONE',  ( 65.00000000000000000, 0.000000000000000000, 0.000000000000000000 ) ) ;
#40121=CARTESIAN_POINT ( 'NONE',  ( 45.00000000000000000, -6.363961030678960462, -6.363961030678893849 ) ) ;
#40152=DIRECTION ( 'NONE',  ( 1.000000000000000000, -0.000000000000000000, -0.000000000000000000 ) ) ;
#40213=VERTEX_POINT ( 'NONE', #49493 ) ;
#40354=ORIENTED_EDGE ( 'NONE', *, *, #30402, .F. ) ;
#40447=VERTEX_POINT ( 'NONE', #52030 ) ;
#40518=ORIENTED_EDGE ( 'NONE', *, *, #35579, .T. ) ;
#40533=ORIENTED_EDGE ( 'NONE', *, *, #13214, .F. ) ;
#40783=AXIS2_PLACEMENT_3D ( 'NONE', #18312, #56413, #39428 ) ;
#40876=DIRECTION ( 'NONE',  ( 1.000000000000000000, 0.000000000000000000, 0.000000000000000000 ) ) ;
#41039=STYLED_ITEM('',(#73144),#21999);
#41205=VERTEX_POINT ( 'NONE', #70428 ) ;
#41236=ORIENTED_EDGE ( 'NONE', *, *, #29224, .F. ) ;
#41428=EDGE_CURVE ( 'NONE', #40447, #48472, #36075, .T. ) ;
#41589=CARTESIAN_POINT ( 'NONE',  ( 20.78732959644809952, 4.500000000000001776, 5.500000000000000000 ) ) ;
#41697=LINE ( 'NONE', #64221, #56090 ) ;
#41796=ORIENTED_EDGE ( 'NONE', *, *, #2338, .F. ) ;
#41912=( NAMED_UNIT ( * ) PLANE_ANGLE_UNIT ( ) SI_UNIT ( $, .RADIAN. ) );
#42308=LINE ( 'NONE', #70381, #64216 ) ;
#42405=CARTESIAN_POINT ( 'NONE',  ( 45.00000000000000000, -2.499999999999999556, -5.500000000000000000 ) ) ;
#42570=EDGE_LOOP ( 'NONE', ( #68240, #42938, #18589, #55019 ) ) ;
#42670=EDGE_CURVE ( 'NONE', #66931, #71147, #26608, .T. ) ;
#42699=CARTESIAN_POINT ( 'NONE',  ( 34.99999999999999289, -2.499999999999999556, -3.499999999999999556 ) ) ;
#42776=CARTESIAN_POINT ( 'NONE',  ( 45.00000000000000000, -4.500000000000000000, 3.499999999999999556 ) ) ;
#42909=ADVANCED_FACE ( 'NONE', ( #54785 ), #31149, .T. ) ;
#42923=ORIENTED_EDGE ( 'NONE', *, *, #26050, .F. ) ;
#42938=ORIENTED_EDGE ( 'NONE', *, *, #14420, .F. ) ;
#43005=VECTOR ( 'NONE', #11283, 1000.000000000000000 ) ;
#43037=AXIS2_PLACEMENT_3D ( 'NONE', #26412, #36400, #37120 ) ;
#43049=CARTESIAN_POINT ( 'NONE',  ( 34.99999999999999289, 6.363961030678916053, -6.363961030678939146 ) ) ;
#43098=CARTESIAN_POINT ( 'NONE',  ( 34.99999999999999289, -6.363961030678871644, 4.863961030678981778 ) ) ;
#43165=AXIS2_PLACEMENT_3D ( 'NONE', #32252, #10089, #3084 ) ;
#43170=CARTESIAN_POINT ( 'NONE',  ( 34.99999999999999289, 6.363961030679004871, 6.363961030678849440 ) ) ;
#43328=DIRECTION ( 'NONE',  ( 0.000000000000000000, 1.000000000000000000, -8.673617379884036705E-17 ) ) ;
#43344=CARTESIAN_POINT ( 'NONE',  ( 50.00000000000000000, -1.494782592887706318, -8.874999999999994671 ) ) ;
#43451=ORIENTED_EDGE ( 'NONE', *, *, #25255, .T. ) ;
#43454=CARTESIAN_POINT ( 'NONE',  ( 20.78732959644809952, -2.499999999999999556, 3.499999999999999556 ) ) ;
#43507=EDGE_CURVE ( 'NONE', #68862, #51352, #63944, .T. ) ;
#43513=DIRECTION ( 'NONE',  ( -1.000000000000000000, -0.000000000000000000, -0.000000000000000000 ) ) ;
#43521=ADVANCED_FACE ( 'NONE', ( #23335 ), #13329, .F. ) ;
#43818=CARTESIAN_POINT ( 'NONE',  ( 45.00000000000000000, -8.874999999999998224, 1.494782592887687667 ) ) ;
#43845=DIRECTION ( 'NONE',  ( 1.000000000000000000, 0.000000000000000000, 0.000000000000000000 ) ) ;
#43855=EDGE_LOOP ( 'NONE', ( #7806, #71888, #16796, #48163, #28104, #15756, #15392, #62455, #188, #61857, #66700, #39366, #53451, #69955, #46717, #68886, #51923, #50278, #23030 ) ) ;
#44057=CARTESIAN_POINT ( 'NONE',  ( 20.78732959644809952, -2.499999999999999556, -3.499999999999999556 ) ) ;
#44114=DIRECTION ( 'NONE',  ( 0.000000000000000000, 0.7071067811865535679, 0.7071067811865414665 ) ) ;
#44158=AXIS2_PLACEMENT_3D ( 'NONE', #33581, #61654, #66480 ) ;
#44223=VERTEX_POINT ( 'NONE', #11461 ) ;
#44238=VECTOR ( 'NONE', #61945, 1000.000000000000000 ) ;
#44270=ORIENTED_EDGE ( 'NONE', *, *, #446, .F. ) ;
#44293=CIRCLE ( 'NONE', #54867, 9.000000000000000000 ) ;
#44325=CIRCLE ( 'NONE', #12443, 1.500000000000000444 ) ;
#44332=CIRCLE ( 'NONE', #40783, 9.000000000000000000 ) ;
#44343=DIRECTION ( 'NONE',  ( 1.000000000000000000, 0.000000000000000000, 0.000000000000000000 ) ) ;
#44378=VECTOR ( 'NONE', #32052, 1000.000000000000000 ) ;
#44429=VECTOR ( 'NONE', #61760, 1000.000000000000000 ) ;
#44443=ORIENTED_EDGE ( 'NONE', *, *, #18286, .T. ) ;
#44487=AXIS2_PLACEMENT_3D ( 'NONE', #70022, #40876, #46774 ) ;
#44620=CARTESIAN_POINT ( 'NONE',  ( 50.00000000000000000, 1.494782592887643924, -8.875000000000003553 ) ) ;
#44714=CARTESIAN_POINT ( 'NONE',  ( 34.99999999999999289, 9.000000000000000000, 0.000000000000000000 ) ) ;
#44755=VERTEX_POINT ( 'NONE', #18431 ) ;
#44872=EDGE_CURVE ( 'NONE', #71649, #57451, #7713, .T. ) ;
#44904=DIRECTION ( 'NONE',  ( 0.000000000000000000, 0.000000000000000000, -1.000000000000000000 ) ) ;
#44990=FACE_BOUND ( 'NONE', #68012, .T. ) ;
#45002=CARTESIAN_POINT ( 'NONE',  ( 20.78732959644809952, -2.499999999999999556, -5.500000000000000000 ) ) ;
#45040=EDGE_CURVE ( 'NONE', #68374, #25347, #20993, .T. ) ;
#45046=CYLINDRICAL_SURFACE ( 'NONE', #44158, 1.500000000000000444 ) ;
#45111=CIRCLE ( 'NONE', #66300, 1.500000000000000444 ) ;
#45144=CARTESIAN_POINT ( 'NONE',  ( 34.99999999999999289, -6.363961030678960462, -6.363961030678893849 ) ) ;
#45328=DIRECTION ( 'NONE',  ( 0.000000000000000000, -1.000000000000000000, 0.000000000000000000 ) ) ;
#45370=AXIS2_PLACEMENT_3D ( 'NONE', #23043, #58828, #13772 ) ;
#45469=EDGE_LOOP ( 'NONE', ( #54998, #24799, #7603, #22935 ) ) ;
#45493=ORIENTED_EDGE ( 'NONE', *, *, #32022, .F. ) ;
#45503=ADVANCED_FACE ( 'NONE', ( #45728 ), #67539, .T. ) ;
#45548=AXIS2_PLACEMENT_3D ( 'NONE', #39728, #15709, #55615 ) ;
#45612=CIRCLE ( 'NONE', #30249, 1.500000000000000444 ) ;
#45638=ADVANCED_FACE ( 'NONE', ( #62706 ), #57152, .T. ) ;
#45652=CARTESIAN_POINT ( 'NONE',  ( 65.00000000000000000, -8.874999999999998224, 1.494782592887675232 ) ) ;
#45728=FACE_OUTER_BOUND ( 'NONE', #60690, .T. ) ;
#45910=CARTESIAN_POINT ( 'NONE',  ( 50.00000000000000000, 5.218601775200110815, -7.332543590861103411 ) ) ;
#46002=ADVANCED_FACE ( 'NONE', ( #19828 ), #57539, .T. ) ;
#46012=DIRECTION ( 'NONE',  ( 1.000000000000000000, 0.000000000000000000, 0.000000000000000000 ) ) ;
#46096=ORIENTED_EDGE ( 'NONE', *, *, #37581, .F. ) ;
#46128=LINE ( 'NONE', #1799, #33544 ) ;
#46259=ORIENTED_EDGE ( 'NONE', *, *, #18286, .F. ) ;
#46294=CARTESIAN_POINT ( 'NONE',  ( 50.00000000000000000, 7.332543590861084759, -5.218601775200136572 ) ) ;
#46307=AXIS2_PLACEMENT_3D ( 'NONE', #48819, #54724, #48088 ) ;
#46370=CARTESIAN_POINT ( 'NONE',  ( 45.00000000000000000, -1.494782592887594852, 8.875000000000012434 ) ) ;
#46605=CARTESIAN_POINT ( 'NONE',  ( 34.99999999999999289, 9.426999614876460059E-14, 9.000000000000000000 ) ) ;
#46627=AXIS2_PLACEMENT_3D ( 'NONE', #65137, #14163, #2011 ) ;
#46717=ORIENTED_EDGE ( 'NONE', *, *, #8966, .T. ) ;
#46759=EDGE_CURVE ( 'NONE', #71649, #54715, #20714, .T. ) ;
#46774=DIRECTION ( 'NONE',  ( 0.000000000000000000, 0.000000000000000000, -1.000000000000000000 ) ) ;
#46789=VERTEX_POINT ( 'NONE', #9854 ) ;
#46801=ORIENTED_EDGE ( 'NONE', *, *, #47241, .F. ) ;
#46820=EDGE_CURVE ( 'NONE', #25475, #38626, #64902, .T. ) ;
#46934=APPLICATION_CONTEXT ( 'automotive_design' ) ;
#47055=CARTESIAN_POINT ( 'NONE',  ( 65.00000000000000000, 9.426999614876460059E-14, 9.000000000000000000 ) ) ;
#47137=ORIENTED_EDGE ( 'NONE', *, *, #1197, .T. ) ;
#47241=EDGE_CURVE ( 'NONE', #39465, #40447, #44325, .T. ) ;
#47282=CARTESIAN_POINT ( 'NONE',  ( 45.00000000000000000, -6.363961030678871644, 4.863961030678981778 ) ) ;
#47360=VERTEX_POINT ( 'NONE', #1681 ) ;
#47404=VECTOR ( 'NONE', #69998, 1000.000000000000000 ) ;
#47560=VERTEX_POINT ( 'NONE', #30104 ) ;
#47565=CARTESIAN_POINT ( 'NONE',  ( 65.00000000000000000, 0.000000000000000000, 0.000000000000000000 ) ) ;
#47643=DIRECTION ( 'NONE',  ( -1.000000000000000000, -0.000000000000000000, -0.000000000000000000 ) ) ;
#47738=CLOSED_SHELL ( 'NONE', ( #63892, #56255, #58996, #51871, #45638, #3977, #34487, #22381, #54331, #46002, #37578, #42909, #45503, #38148, #50000, #70271, #1478, #70933, #72125, #12590, #28872, #28309, #29071, #27330, #1080, #27821, #43521, #71684, #61479, #35138, #31836 ) ) ;
#47842=AXIS2_PLACEMENT_3D ( 'NONE', #13928, #69003, #35731 ) ;
#47847=AXIS2_PLACEMENT_3D ( 'NONE', #32177, #66522, #49179 ) ;
#47892=DIRECTION ( 'NONE',  ( -1.000000000000000000, -0.000000000000000000, -0.000000000000000000 ) ) ;
#47949=DIRECTION ( 'NONE',  ( 0.000000000000000000, 1.000000000000000000, -8.673617379884036705E-17 ) ) ;
#48020=CARTESIAN_POINT ( 'NONE',  ( 65.00000000000000000, 0.000000000000000000, 0.000000000000000000 ) ) ;
#48088=DIRECTION ( 'NONE',  ( 0.000000000000000000, 0.000000000000000000, -1.000000000000000000 ) ) ;
#48163=ORIENTED_EDGE ( 'NONE', *, *, #47241, .T. ) ;
#48229=FACE_OUTER_BOUND ( 'NONE', #55691, .T. ) ;
#48416=DIRECTION ( 'NONE',  ( 0.000000000000000000, 1.000000000000000000, -8.673617379884036705E-17 ) ) ;
#48448=VERTEX_POINT ( 'NONE', #6766 ) ;
#48472=VERTEX_POINT ( 'NONE', #30386 ) ;
#48610=ORIENTED_EDGE ( 'NONE', *, *, #54938, .T. ) ;
#48625=DIRECTION ( 'NONE',  ( 0.000000000000000000, -1.000000000000000000, 0.000000000000000000 ) ) ;
#48642=AXIS2_PLACEMENT_3D ( 'NONE', #30883, #14618, #20153 ) ;
#48764=EDGE_LOOP ( 'NONE', ( #27818, #10404, #34786, #46096 ) ) ;
#48819=CARTESIAN_POINT ( 'NONE',  ( 34.99999999999999289, -6.363961030678871644, 6.363961030678982667 ) ) ;
#48922=DIRECTION ( 'NONE',  ( 1.000000000000000000, 0.000000000000000000, 0.000000000000000000 ) ) ;
#48977=ORIENTED_EDGE ( 'NONE', *, *, #32022, .T. ) ;
#49034=AXIS2_PLACEMENT_3D ( 'NONE', #46605, #17778, #1549 ) ;
#49053=PLANE ( 'NONE',  #60849 ) ;
#49099=ORIENTED_EDGE ( 'NONE', *, *, #25255, .F. ) ;
#49179=DIRECTION ( 'NONE',  ( 0.000000000000000000, 0.000000000000000000, -1.000000000000000000 ) ) ;
#49235=DIRECTION ( 'NONE',  ( 0.000000000000000000, -8.673617379884036705E-17, -1.000000000000000000 ) ) ;
#49314=CIRCLE ( 'NONE', #17427, 1.500000000000000444 ) ;
#49413=DIRECTION ( 'NONE',  ( 0.000000000000000000, -1.000000000000000000, 3.469446951953613006E-15 ) ) ;
#49493=CARTESIAN_POINT ( 'NONE',  ( 65.00000000000000000, -6.363961030678871644, 4.863961030678981778 ) ) ;
#49496=CARTESIAN_POINT ( 'NONE',  ( 65.00000000000000000, 1.494782592887768269, 8.874999999999982236 ) ) ;
#49612=DIRECTION ( 'NONE',  ( 0.000000000000000000, 0.000000000000000000, 1.000000000000000000 ) ) ;
#49669=EDGE_CURVE ( 'NONE', #33507, #19228, #14866, .T. ) ;
#49704=DIRECTION ( 'NONE',  ( 0.000000000000000000, 0.7071067811865535679, 0.7071067811865414665 ) ) ;
#49711=ORIENTED_EDGE ( 'NONE', *, *, #58454, .F. ) ;
#49752=CARTESIAN_POINT ( 'NONE',  ( 65.00000000000000000, 6.363961030678916053, -6.363961030678939146 ) ) ;
#49778=DIRECTION ( 'NONE',  ( 1.000000000000000000, -0.000000000000000000, -0.000000000000000000 ) ) ;
#49845=ORIENTED_EDGE ( 'NONE', *, *, #49856, .T. ) ;
#49856=EDGE_CURVE ( 'NONE', #33629, #29982, #21321, .T. ) ;
#49871=CARTESIAN_POINT ( 'NONE',  ( 45.00000000000000000, -2.499999999999999556, 3.499999999999999556 ) ) ;
#50000=ADVANCED_FACE ( 'NONE', ( #14680 ), #49053, .F. ) ;
#50084=ORIENTED_EDGE ( 'NONE', *, *, #45040, .F. ) ;
#50150=LINE ( 'NONE', #44620, #44238 ) ;
#50183=DIRECTION ( 'NONE',  ( -1.000000000000000000, -0.000000000000000000, -0.000000000000000000 ) ) ;
#50193=ORIENTED_EDGE ( 'NONE', *, *, #68511, .F. ) ;
#50278=ORIENTED_EDGE ( 'NONE', *, *, #21587, .F. ) ;
#50363=DIRECTION ( 'NONE',  ( 1.000000000000000000, 0.000000000000000000, 0.000000000000000000 ) ) ;
#50445=CARTESIAN_POINT ( 'NONE',  ( 45.00000000000000000, 7.332543590861163807, 5.218601775200022885 ) ) ;
#50552=ORIENTED_EDGE ( 'NONE', *, *, #24944, .T. ) ;
#50774=CARTESIAN_POINT ( 'NONE',  ( 50.00000000000000000, -1.494782592887582195, 8.875000000000014211 ) ) ;
#50799=EDGE_LOOP ( 'NONE', ( #19042, #36110, #21698, #4198 ) ) ;
#50800=DIRECTION ( 'NONE',  ( 1.000000000000000000, 0.000000000000000000, 0.000000000000000000 ) ) ;
#50924=EDGE_CURVE ( 'NONE', #46789, #56113, #67681, .T. ) ;
#51061=CARTESIAN_POINT ( 'NONE',  ( 45.00000000000000000, 2.500000000000000444, 5.500000000000000000 ) ) ;
#51287=CIRCLE ( 'NONE', #45548, 9.000000000000000000 ) ;
#51352=VERTEX_POINT ( 'NONE', #7405 ) ;
#51480=DIRECTION ( 'NONE',  ( 1.000000000000000000, 0.000000000000000000, 0.000000000000000000 ) ) ;
#51513=DIRECTION ( 'NONE',  ( 0.000000000000000000, 0.000000000000000000, -1.000000000000000000 ) ) ;
#51564=ORIENTED_EDGE ( 'NONE', *, *, #18886, .T. ) ;
#51598=FACE_OUTER_BOUND ( 'NONE', #48764, .T. ) ;
#51604=ORIENTED_EDGE ( 'NONE', *, *, #12260, .T. ) ;
#51755=VERTEX_POINT ( 'NONE', #47282 ) ;
#51786=DIRECTION ( 'NONE',  ( 1.000000000000000000, -0.000000000000000000, -0.000000000000000000 ) ) ;
#51796=CYLINDRICAL_SURFACE ( 'NONE', #20614, 9.000000000000000000 ) ;
#51871=ADVANCED_FACE ( 'NONE', ( #9220 ), #8482, .T. ) ;
#51923=ORIENTED_EDGE ( 'NONE', *, *, #68367, .T. ) ;
#52030=CARTESIAN_POINT ( 'NONE',  ( 45.00000000000000000, -7.332543590861129168, -5.218601775200074400 ) ) ;
#52040=DIRECTION ( 'NONE',  ( 0.000000000000000000, 0.000000000000000000, -1.000000000000000000 ) ) ;
#52158=CIRCLE ( 'NONE', #63957, 1.500000000000000444 ) ;
#52369=CARTESIAN_POINT ( 'NONE',  ( 45.00000000000000000, -4.500000000000000000, 5.500000000000000888 ) ) ;
#52660=CIRCLE ( 'NONE', #66866, 9.000000000000000000 ) ;
#52725=CARTESIAN_POINT ( 'NONE',  ( 45.00000000000000000, -6.363961030678871644, 6.363961030678982667 ) ) ;
#52738=ORIENTED_EDGE ( 'NONE', *, *, #4935, .F. ) ;
#53035=CARTESIAN_POINT ( 'NONE',  ( 45.00000000000000000, -7.332543590861054561, 5.218601775200177428 ) ) ;
#53058=CARTESIAN_POINT ( 'NONE',  ( 65.00000000000000000, -1.494782592887582195, 8.875000000000012434 ) ) ;
#53123=CARTESIAN_POINT ( 'NONE',  ( 20.78732959644809952, 2.500000000000000444, 5.500000000000000000 ) ) ;
#53155=LINE ( 'NONE', #2553, #1997 ) ;
#53357=( LENGTH_UNIT ( ) NAMED_UNIT ( * ) SI_UNIT ( .MILLI., .METRE. ) );
#53391=VECTOR ( 'NONE', #13314, 1000.000000000000000 ) ;
#53451=ORIENTED_EDGE ( 'NONE', *, *, #3140, .F. ) ;
#53471=CARTESIAN_POINT ( 'NONE',  ( 65.00000000000000000, 5.218601775200212955, 7.332543590861030580 ) ) ;
#53473=DIRECTION ( 'NONE',  ( 0.000000000000000000, 0.000000000000000000, -1.000000000000000000 ) ) ;
#53687=AXIS2_PLACEMENT_3D ( 'NONE', #43049, #70753, #20128 ) ;
#53756=VECTOR ( 'NONE', #12784, 1000.000000000000000 ) ;
#53797=CARTESIAN_POINT ( 'NONE',  ( 45.00000000000000000, 0.000000000000000000, 0.000000000000000000 ) ) ;
#53820=CYLINDRICAL_SURFACE ( 'NONE', #21839, 1.500000000000000444 ) ;
#53867=FACE_OUTER_BOUND ( 'NONE', #10378, .T. ) ;
#53958=LINE ( 'NONE', #60569, #20568 ) ;
#54009=CARTESIAN_POINT ( 'NONE',  ( 65.00000000000000000, 8.874999999999998224, -1.494782592887675232 ) ) ;
#54047=AXIS2_PLACEMENT_3D ( 'NONE', #19670, #69930, #58101 ) ;
#54059=VERTEX_POINT ( 'NONE', #58287 ) ;
#54116=ADVANCED_BREP_SHAPE_REPRESENTATION ( '', ( #21999, #23765 ), #19014 ) ;
#54143=EDGE_LOOP ( 'NONE', ( #31299, #11129, #72606, #22351 ) ) ;
#54331=ADVANCED_FACE ( 'NONE', ( #20958 ), #31692, .T. ) ;
#54392=VERTEX_POINT ( 'NONE', #32057 ) ;
#54418=ORIENTED_EDGE ( 'NONE', *, *, #9015, .T. ) ;
#54436=DIRECTION ( 'NONE',  ( 0.000000000000000000, 0.000000000000000000, -1.000000000000000000 ) ) ;
#54504=ORIENTED_EDGE ( 'NONE', *, *, #65415, .F. ) ;
#54515=DIRECTION ( 'NONE',  ( 0.000000000000000000, 1.000000000000000000, -8.673617379884036705E-17 ) ) ;
#54715=VERTEX_POINT ( 'NONE', #72309 ) ;
#54724=DIRECTION ( 'NONE',  ( 1.000000000000000000, -0.000000000000000000, -0.000000000000000000 ) ) ;
#54740=ORIENTED_EDGE ( 'NONE', *, *, #34570, .F. ) ;
#54785=FACE_OUTER_BOUND ( 'NONE', #14201, .T. ) ;
#54867=AXIS2_PLACEMENT_3D ( 'NONE', #6440, #21974, #51513 ) ;
#54938=EDGE_CURVE ( 'NONE', #39465, #54059, #22049, .T. ) ;
#54998=ORIENTED_EDGE ( 'NONE', *, *, #30954, .T. ) ;
#55019=ORIENTED_EDGE ( 'NONE', *, *, #33157, .T. ) ;
#55154=FACE_OUTER_BOUND ( 'NONE', #67073, .T. ) ;
#55166=VERTEX_POINT ( 'NONE', #12064 ) ;
#55175=DIRECTION ( 'NONE',  ( 1.000000000000000000, 0.000000000000000000, 0.000000000000000000 ) ) ;
#55385=VERTEX_POINT ( 'NONE', #20492 ) ;
#55487=ORIENTED_EDGE ( 'NONE', *, *, #13371, .F. ) ;
#55514=ORIENTED_EDGE ( 'NONE', *, *, #11404, .T. ) ;
#55612=ORIENTED_EDGE ( 'NONE', *, *, #32061, .T. ) ;
#55615=DIRECTION ( 'NONE',  ( 0.000000000000000000, 0.000000000000000000, -1.000000000000000000 ) ) ;
#55654=DIRECTION ( 'NONE',  ( 1.000000000000000000, -0.000000000000000000, -0.000000000000000000 ) ) ;
#55691=EDGE_LOOP ( 'NONE', ( #40533, #73061, #21170, #55487 ) ) ;
#55695=EDGE_LOOP ( 'NONE', ( #50084, #48977, #15706, #46259 ) ) ;
#55777=DIRECTION ( 'NONE',  ( 0.000000000000000000, 0.000000000000000000, -1.000000000000000000 ) ) ;
#55898=DIRECTION ( 'NONE',  ( 0.000000000000000000, 0.000000000000000000, -1.000000000000000000 ) ) ;
#55907=CARTESIAN_POINT ( 'NONE',  ( 45.00000000000000000, 6.363961030678916053, -6.363961030678939146 ) ) ;
#55933=DIRECTION ( 'NONE',  ( 1.000000000000000000, 0.000000000000000000, 0.000000000000000000 ) ) ;
#55980=LINE ( 'NONE', #5374, #43005 ) ;
#56041=DIRECTION ( 'NONE',  ( 1.000000000000000000, 0.000000000000000000, 0.000000000000000000 ) ) ;
#56090=VECTOR ( 'NONE', #18058, 1000.000000000000000 ) ;
#56113=VERTEX_POINT ( 'NONE', #49496 ) ;
#56116=DIRECTION ( 'NONE',  ( 0.000000000000000000, 0.000000000000000000, -1.000000000000000000 ) ) ;
#56251=ORIENTED_EDGE ( 'NONE', *, *, #68367, .F. ) ;
#56255=ADVANCED_FACE ( 'NONE', ( #22496 ), #45046, .F. ) ;
#56317=VECTOR ( 'NONE', #16733, 1000.000000000000000 ) ;
#56370=CARTESIAN_POINT ( 'NONE',  ( 45.00000000000000000, -5.218601775200152559, -7.332543590861073213 ) ) ;
#56402=DIRECTION ( 'NONE',  ( 0.000000000000000000, 0.7071067811865388020, -0.7071067811865562325 ) ) ;
#56413=DIRECTION ( 'NONE',  ( 1.000000000000000000, 0.000000000000000000, 0.000000000000000000 ) ) ;
#56475=EDGE_CURVE ( 'NONE', #55166, #39465, #46128, .T. ) ;
#56528=ORIENTED_EDGE ( 'NONE', *, *, #68511, .T. ) ;
#56652=LINE ( 'NONE', #6410, #39520 ) ;
#56894=ORIENTED_EDGE ( 'NONE', *, *, #2674, .F. ) ;
#56931=LINE ( 'NONE', #23315, #12356 ) ;
#56945=EDGE_LOOP ( 'NONE', ( #71357, #71957, #10315, #61384 ) ) ;
#57084=DIRECTION ( 'NONE',  ( 0.000000000000000000, 0.000000000000000000, -1.000000000000000000 ) ) ;
#57152=CYLINDRICAL_SURFACE ( 'NONE', #70239, 9.000000000000000000 ) ;
#57160=ORIENTED_EDGE ( 'NONE', *, *, #60001, .T. ) ;
#57194=DIRECTION ( 'NONE',  ( -1.000000000000000000, -0.000000000000000000, 0.000000000000000000 ) ) ;
#57263=VECTOR ( 'NONE', #59413, 1000.000000000000000 ) ;
#57285=UNCERTAINTY_MEASURE_WITH_UNIT (LENGTH_MEASURE( 1.000000000000000082E-05 ), #53357, 'distance_accuracy_value', 'NONE');
#57451=VERTEX_POINT ( 'NONE', #54009 ) ;
#57539=CYLINDRICAL_SURFACE ( 'NONE', #47842, 9.000000000000000000 ) ;
#57569=DIRECTION ( 'NONE',  ( 0.000000000000000000, 0.000000000000000000, -1.000000000000000000 ) ) ;
#57824=EDGE_CURVE ( 'NONE', #44223, #44755, #6936, .T. ) ;
#57843=LINE ( 'NONE', #28694, #53756 ) ;
#57851=ORIENTED_EDGE ( 'NONE', *, *, #8189, .T. ) ;
#58101=DIRECTION ( 'NONE',  ( 0.000000000000000000, 0.000000000000000000, -1.000000000000000000 ) ) ;
#58263=ORIENTED_EDGE ( 'NONE', *, *, #61088, .F. ) ;
#58268=FACE_OUTER_BOUND ( 'NONE', #20666, .T. ) ;
#58287=CARTESIAN_POINT ( 'NONE',  ( 45.00000000000000000, -1.494782592887718531, -8.874999999999992895 ) ) ;
#58303=CARTESIAN_POINT ( 'NONE',  ( 65.00000000000000000, 9.426999614876460059E-14, 7.499999999999999112 ) ) ;
#58306=DIRECTION ( 'NONE',  ( 1.000000000000000000, 0.000000000000000000, -0.000000000000000000 ) ) ;
#58366=AXIS2_PLACEMENT_3D ( 'NONE', #31991, #47892, #30886 ) ;
#58454=EDGE_CURVE ( 'NONE', #44755, #8380, #26881, .T. ) ;
#58610=FACE_OUTER_BOUND ( 'NONE', #15536, .T. ) ;
#58828=DIRECTION ( 'NONE',  ( 1.000000000000000000, 0.000000000000000000, 0.000000000000000000 ) ) ;
#58926=ORIENTED_EDGE ( 'NONE', *, *, #65415, .T. ) ;
#58930=PRODUCT_DEFINITION ( 'UNKNOWN', '', #9662, #24025 ) ;
#58996=ADVANCED_FACE ( 'NONE', ( #67854 ), #62303, .F. ) ;
#59108=EDGE_CURVE ( 'NONE', #51352, #70677, #35848, .T. ) ;
#59147=FACE_OUTER_BOUND ( 'NONE', #42570, .T. ) ;
#59156=VERTEX_POINT ( 'NONE', #5432 ) ;
#59309=CARTESIAN_POINT ( 'NONE',  ( 34.99999999999999289, 2.500000000000000444, 3.499999999999999112 ) ) ;
#59334=DIRECTION ( 'NONE',  ( 1.000000000000000000, -0.000000000000000000, -0.000000000000000000 ) ) ;
#59413=DIRECTION ( 'NONE',  ( 0.000000000000000000, -1.000000000000000000, 8.673617379884035472E-17 ) ) ;
#59513=CARTESIAN_POINT ( 'NONE',  ( 65.00000000000000000, 7.332543590861083871, -5.218601775200134796 ) ) ;
#59649=DIRECTION ( 'NONE',  ( -1.000000000000000000, 0.000000000000000000, 0.000000000000000000 ) ) ;
#59686=FACE_OUTER_BOUND ( 'NONE', #34877, .T. ) ;
#59690=DIRECTION ( 'NONE',  ( 0.000000000000000000, -0.000000000000000000, -1.000000000000000000 ) ) ;
#59897=EDGE_CURVE ( 'NONE', #10639, #51352, #33590, .T. ) ;
#59934=( NAMED_UNIT ( * ) PLANE_ANGLE_UNIT ( ) SI_UNIT ( $, .RADIAN. ) );
#60001=EDGE_CURVE ( 'NONE', #15065, #41205, #42308, .T. ) ;
#60203=LINE ( 'NONE', #49871, #26499 ) ;
#60259=VERTEX_POINT ( 'NONE', #27152 ) ;
#60310=COLOUR_RGB ( '',0.8941176470588234615, 0.8941176470588234615, 0.8941176470588234615 ) ;
#60347=SHAPE_DEFINITION_REPRESENTATION ( #11961, #68023 ) ;
#60394=CARTESIAN_POINT ( 'NONE',  ( 65.00000000000000000, -6.363961030678871644, 6.363961030678982667 ) ) ;
#60569=CARTESIAN_POINT ( 'NONE',  ( 45.00000000000000000, -2.499999999999999556, -3.499999999999999556 ) ) ;
#60675=CARTESIAN_POINT ( 'NONE',  ( 20.78732959644809952, 4.500000000000000888, -3.500000000000000000 ) ) ;
#60690=EDGE_LOOP ( 'NONE', ( #30710, #40518, #55514, #49711 ) ) ;
#60749=AXIS2_PLACEMENT_3D ( 'NONE', #44057, #49235, #43328 ) ;
#60849=AXIS2_PLACEMENT_3D ( 'NONE', #10612, #20217, #5076 ) ;
#60868=CARTESIAN_POINT ( 'NONE',  ( 20.78732959644809952, -2.499999999999999556, 3.499999999999999556 ) ) ;
#61050=AXIS2_PLACEMENT_3D ( 'NONE', #30563, #64535, #13193 ) ;
#61088=EDGE_CURVE ( 'NONE', #25347, #68777, #71024, .T. ) ;
#61384=ORIENTED_EDGE ( 'NONE', *, *, #32153, .F. ) ;
#61479=ADVANCED_FACE ( 'NONE', ( #6617 ), #18037, .F. ) ;
#61543=CARTESIAN_POINT ( 'NONE',  ( 45.00000000000000000, 6.363961030679004871, 6.363961030678849440 ) ) ;
#61654=DIRECTION ( 'NONE',  ( 1.000000000000000000, -0.000000000000000000, -0.000000000000000000 ) ) ;
#61665=EDGE_CURVE ( 'NONE', #72600, #68862, #72519, .T. ) ;
#61760=DIRECTION ( 'NONE',  ( 1.000000000000000000, -0.000000000000000000, -0.000000000000000000 ) ) ;
#61840=EDGE_CURVE ( 'NONE', #55166, #48472, #26534, .T. ) ;
#61857=ORIENTED_EDGE ( 'NONE', *, *, #6767, .F. ) ;
#61916=LINE ( 'NONE', #22393, #64345 ) ;
#61936=VECTOR ( 'NONE', #40152, 1000.000000000000000 ) ;
#61945=DIRECTION ( 'NONE',  ( -1.000000000000000000, -0.000000000000000000, 0.000000000000000000 ) ) ;
#61967=DIRECTION ( 'NONE',  ( 0.000000000000000000, 0.000000000000000000, -1.000000000000000000 ) ) ;
#61974=DIRECTION ( 'NONE',  ( 0.000000000000000000, 0.000000000000000000, -1.000000000000000000 ) ) ;
#61989=AXIS2_PLACEMENT_3D ( 'NONE', #60675, #26720, #36690 ) ;
#62018=ORIENTED_EDGE ( 'NONE', *, *, #61665, .F. ) ;
#62022=AXIS2_PLACEMENT_3D ( 'NONE', #49752, #43845, #9492 ) ;
#62031=AXIS2_PLACEMENT_3D ( 'NONE', #38526, #27081, #49612 ) ;
#62303=CYLINDRICAL_SURFACE ( 'NONE', #70089, 1.500000000000000444 ) ;
#62455=ORIENTED_EDGE ( 'NONE', *, *, #14420, .T. ) ;
#62575=EDGE_CURVE ( 'NONE', #10639, #72600, #64239, .T. ) ;
#62706=FACE_OUTER_BOUND ( 'NONE', #4729, .T. ) ;
#62734=ORIENTED_EDGE ( 'NONE', *, *, #65317, .T. ) ;
#63093=ORIENTED_EDGE ( 'NONE', *, *, #6767, .T. ) ;
#63305=AXIS2_PLACEMENT_3D ( 'NONE', #67569, #33931, #56116 ) ;
#63425=CARTESIAN_POINT ( 'NONE',  ( 45.00000000000000000, 4.500000000000000888, -5.500000000000000888 ) ) ;
#63812=ORIENTED_EDGE ( 'NONE', *, *, #22708, .T. ) ;
#63892=ADVANCED_FACE ( 'NONE', ( #58610 ), #53820, .F. ) ;
#63903=( GEOMETRIC_REPRESENTATION_CONTEXT ( 3 ) GLOBAL_UNCERTAINTY_ASSIGNED_CONTEXT ( ( #3340 ) ) GLOBAL_UNIT_ASSIGNED_CONTEXT ( ( #12739, #3861, #71824 ) ) REPRESENTATION_CONTEXT ( 'NONE', 'WORKASPACE' ) );
#63944=LINE ( 'NONE', #23694, #19508 ) ;
#63957=AXIS2_PLACEMENT_3D ( 'NONE', #8354, #14988, #64131 ) ;
#64043=CARTESIAN_POINT ( 'NONE',  ( 34.99999999999999289, -2.499999999999999556, 3.499999999999999556 ) ) ;
#64072=LINE ( 'NONE', #25657, #26896 ) ;
#64131=DIRECTION ( 'NONE',  ( 0.000000000000000000, 0.000000000000000000, -1.000000000000000000 ) ) ;
#64200=CARTESIAN_POINT ( 'NONE',  ( 65.00000000000000000, 0.000000000000000000, 0.000000000000000000 ) ) ;
#64216=VECTOR ( 'NONE', #59649, 1000.000000000000000 ) ;
#64221=CARTESIAN_POINT ( 'NONE',  ( 20.78732959644809952, 2.500000000000000444, 3.499999999999999112 ) ) ;
#64237=EDGE_CURVE ( 'NONE', #51755, #40213, #10937, .T. ) ;
#64239=LINE ( 'NONE', #8100, #38339 ) ;
#64284=CIRCLE ( 'NONE', #6514, 1.500000000000000444 ) ;
#64296=DIRECTION ( 'NONE',  ( 0.000000000000000000, 0.000000000000000000, 1.000000000000000000 ) ) ;
#64345=VECTOR ( 'NONE', #55654, 1000.000000000000000 ) ;
#64437=PRESENTATION_STYLE_ASSIGNMENT (( #69985 ) ) ;
#64511=DIRECTION ( 'NONE',  ( 1.000000000000000000, 0.000000000000000000, -0.000000000000000000 ) ) ;
#64526=VERTEX_POINT ( 'NONE', #46370 ) ;
#64535=DIRECTION ( 'NONE',  ( 1.000000000000000000, 0.000000000000000000, 0.000000000000000000 ) ) ;
#64802=( NAMED_UNIT ( * ) SI_UNIT ( $, .STERADIAN. ) SOLID_ANGLE_UNIT ( ) );
#64816=LINE ( 'NONE', #26030, #47404 ) ;
#64902=LINE ( 'NONE', #36830, #66737 ) ;
#64912=ORIENTED_EDGE ( 'NONE', *, *, #2338, .T. ) ;
#65137=CARTESIAN_POINT ( 'NONE',  ( 65.00000000000000000, -9.000000000000000000, 0.000000000000000000 ) ) ;
#65168=SHAPE_REPRESENTATION_RELATIONSHIP ( 'NONE' , 'NONE' ,  #68023, #54116 ) ;
#65253=DIRECTION ( 'NONE',  ( 0.000000000000000000, 0.000000000000000000, -1.000000000000000000 ) ) ;
#65317=EDGE_CURVE ( 'NONE', #40213, #25827, #12400, .T. ) ;
#65364=DIRECTION ( 'NONE',  ( 0.000000000000000000, 0.000000000000000000, -1.000000000000000000 ) ) ;
#65390=DIRECTION ( 'NONE',  ( 0.000000000000000000, 0.000000000000000000, -1.000000000000000000 ) ) ;
#65415=EDGE_CURVE ( 'NONE', #36937, #68374, #4229, .T. ) ;
#65444=AXIS2_PLACEMENT_3D ( 'NONE', #28064, #28773, #57569 ) ;
#65506=AXIS2_PLACEMENT_3D ( 'NONE', #33361, #31905, #55898 ) ;
#65551=CARTESIAN_POINT ( 'NONE',  ( 45.00000000000000000, 9.426999614876460059E-14, 9.000000000000000000 ) ) ;
#65592=LINE ( 'NONE', #42699, #33665 ) ;
#65603=DIRECTION ( 'NONE',  ( 0.000000000000000000, 0.000000000000000000, -1.000000000000000000 ) ) ;
#65819=ORIENTED_EDGE ( 'NONE', *, *, #14679, .T. ) ;
#65866=DIRECTION ( 'NONE',  ( 1.000000000000000000, 0.000000000000000000, -0.000000000000000000 ) ) ;
#66032=CARTESIAN_POINT ( 'NONE',  ( 20.78732959644809952, -4.500000000000000000, 5.500000000000000888 ) ) ;
#66045=ORIENTED_EDGE ( 'NONE', *, *, #35732, .T. ) ;
#66100=CARTESIAN_POINT ( 'NONE',  ( 45.00000000000000000, 9.426999614876460059E-14, 9.000000000000000000 ) ) ;
#66233=AXIS2_PLACEMENT_3D ( 'NONE', #38462, #33639, #5207 ) ;
#66300=AXIS2_PLACEMENT_3D ( 'NONE', #65551, #55933, #27870 ) ;
#66404=DIRECTION ( 'NONE',  ( 0.000000000000000000, 0.000000000000000000, 1.000000000000000000 ) ) ;
#66480=DIRECTION ( 'NONE',  ( 0.000000000000000000, 0.000000000000000000, -1.000000000000000000 ) ) ;
#66522=DIRECTION ( 'NONE',  ( 1.000000000000000000, 0.000000000000000000, 0.000000000000000000 ) ) ;
#66582=CYLINDRICAL_SURFACE ( 'NONE', #71319, 1.500000000000000444 ) ;
#66677=VECTOR ( 'NONE', #44904, 1000.000000000000000 ) ;
#66700=ORIENTED_EDGE ( 'NONE', *, *, #9386, .T. ) ;
#66718=EDGE_CURVE ( 'NONE', #47560, #17531, #64816, .T. ) ;
#66737=VECTOR ( 'NONE', #32383, 1000.000000000000000 ) ;
#66752=AXIS2_PLACEMENT_3D ( 'NONE', #23612, #58306, #19512 ) ;
#66774=DIRECTION ( 'NONE',  ( 1.000000000000000000, 0.000000000000000000, 0.000000000000000000 ) ) ;
#66866=AXIS2_PLACEMENT_3D ( 'NONE', #69435, #50363, #122 ) ;
#66881=DIRECTION ( 'NONE',  ( 1.000000000000000000, -0.000000000000000000, -0.000000000000000000 ) ) ;
#66931=VERTEX_POINT ( 'NONE', #4245 ) ;
#66975=DIRECTION ( 'NONE',  ( 0.000000000000000000, -1.000000000000000000, 8.673617379884035472E-17 ) ) ;
#67073=EDGE_LOOP ( 'NONE', ( #63093, #51604, #5634, #36043 ) ) ;
#67078=CARTESIAN_POINT ( 'NONE',  ( 34.99999999999999289, -4.500000000000000000, 3.499999999999999556 ) ) ;
#67227=EDGE_CURVE ( 'NONE', #47560, #46789, #45111, .T. ) ;
#67250=DIRECTION ( 'NONE',  ( 0.000000000000000000, 0.000000000000000000, -1.000000000000000000 ) ) ;
#67325=FACE_OUTER_BOUND ( 'NONE', #5322, .T. ) ;
#67370=DIRECTION ( 'NONE',  ( 1.000000000000000000, 0.000000000000000000, 0.000000000000000000 ) ) ;
#67516=ORIENTED_EDGE ( 'NONE', *, *, #33822, .T. ) ;
#67528=PLANE ( 'NONE',  #21857 ) ;
#67539=PLANE ( 'NONE',  #23040 ) ;
#67566=ORIENTED_EDGE ( 'NONE', *, *, #66718, .F. ) ;
#67569=CARTESIAN_POINT ( 'NONE',  ( 45.00000000000000000, -3.142333204958820020E-14, -9.000000000000000000 ) ) ;
#67636=EDGE_CURVE ( 'NONE', #71649, #12198, #23746, .T. ) ;
#67681=LINE ( 'NONE', #22243, #44429 ) ;
#67697=ORIENTED_EDGE ( 'NONE', *, *, #32153, .T. ) ;
#67854=FACE_OUTER_BOUND ( 'NONE', #56945, .T. ) ;
#67864=DIRECTION ( 'NONE',  ( 0.000000000000000000, -0.000000000000000000, -1.000000000000000000 ) ) ;
#68012=EDGE_LOOP ( 'NONE', ( #66045, #24918, #29901, #24480 ) ) ;
#68023=SHAPE_REPRESENTATION ( 'knob', ( #23765 ), #19014 ) ;
#68133=AXIS2_PLACEMENT_3D ( 'NONE', #40013, #67370, #39655 ) ;
#68148=CARTESIAN_POINT ( 'NONE',  ( 20.78732959644809952, 2.500000000000000000, -3.500000000000000000 ) ) ;
#68190=DIRECTION ( 'NONE',  ( 0.000000000000000000, 0.000000000000000000, 1.000000000000000000 ) ) ;
#68221=( GEOMETRIC_REPRESENTATION_CONTEXT ( 3 ) GLOBAL_UNCERTAINTY_ASSIGNED_CONTEXT ( ( #1886 ) ) GLOBAL_UNIT_ASSIGNED_CONTEXT ( ( #37411, #59934, #27067 ) ) REPRESENTATION_CONTEXT ( 'NONE', 'WORKASPACE' ) );
#68240=ORIENTED_EDGE ( 'NONE', *, *, #64237, .F. ) ;
#68367=EDGE_CURVE ( 'NONE', #41205, #59156, #52158, .T. ) ;
#68374=VERTEX_POINT ( 'NONE', #59309 ) ;
#68447=ORIENTED_EDGE ( 'NONE', *, *, #49669, .T. ) ;
#68472=VERTEX_POINT ( 'NONE', #70046 ) ;
#68511=EDGE_CURVE ( 'NONE', #55166, #19228, #7332, .T. ) ;
#68749=ORIENTED_EDGE ( 'NONE', *, *, #30772, .F. ) ;
#68777=VERTEX_POINT ( 'NONE', #36814 ) ;
#68862=VERTEX_POINT ( 'NONE', #25507 ) ;
#68886=ORIENTED_EDGE ( 'NONE', *, *, #8189, .F. ) ;
#68982=CARTESIAN_POINT ( 'NONE',  ( 45.00000000000000000, -5.218601775200048642, 7.332543590861146932 ) ) ;
#69001=DIRECTION ( 'NONE',  ( 1.000000000000000000, 0.000000000000000000, 0.000000000000000000 ) ) ;
#69003=DIRECTION ( 'NONE',  ( -1.000000000000000000, -0.000000000000000000, -0.000000000000000000 ) ) ;
#69016=ORIENTED_EDGE ( 'NONE', *, *, #11404, .F. ) ;
#69060=EDGE_CURVE ( 'NONE', #66931, #40447, #72269, .T. ) ;
#69271=FILL_AREA_STYLE_COLOUR ( '', #60310 ) ;
#69321=ORIENTED_EDGE ( 'NONE', *, *, #59108, .F. ) ;
#69325=ORIENTED_EDGE ( 'NONE', *, *, #46759, .F. ) ;
#69341=CIRCLE ( 'NONE', #37489, 9.000000000000000000 ) ;
#69368=DIRECTION ( 'NONE',  ( 1.000000000000000000, 0.000000000000000000, 0.000000000000000000 ) ) ;
#69382=ORIENTED_EDGE ( 'NONE', *, *, #22708, .F. ) ;
#69435=CARTESIAN_POINT ( 'NONE',  ( 65.00000000000000000, 0.000000000000000000, 0.000000000000000000 ) ) ;
#69923=AXIS2_PLACEMENT_3D ( 'NONE', #38420, #44343, #55777 ) ;
#69930=DIRECTION ( 'NONE',  ( 1.000000000000000000, 0.000000000000000000, 0.000000000000000000 ) ) ;
#69955=ORIENTED_EDGE ( 'NONE', *, *, #61665, .T. ) ;
#69985=SURFACE_STYLE_USAGE ( .BOTH. , #30465 ) ;
#69998=DIRECTION ( 'NONE',  ( 1.000000000000000000, -0.000000000000000000, -0.000000000000000000 ) ) ;
#70022=CARTESIAN_POINT ( 'NONE',  ( 45.00000000000000000, 0.000000000000000000, 0.000000000000000000 ) ) ;
#70046=CARTESIAN_POINT ( 'NONE',  ( 65.00000000000000000, -8.874999999999998224, -1.494782592887675232 ) ) ;
#70089=AXIS2_PLACEMENT_3D ( 'NONE', #17582, #49778, #5792 ) ;
#70239=AXIS2_PLACEMENT_3D ( 'NONE', #6563, #50183, #72711 ) ;
#70271=ADVANCED_FACE ( 'NONE', ( #5721 ), #16425, .F. ) ;
#70381=CARTESIAN_POINT ( 'NONE',  ( 50.00000000000000000, 8.875000000000000000, 1.494782592887675232 ) ) ;
#70428=CARTESIAN_POINT ( 'NONE',  ( 45.00000000000000000, 8.874999999999998224, 1.494782592887687667 ) ) ;
#70492=MECHANICAL_DESIGN_GEOMETRIC_PRESENTATION_REPRESENTATION('',(#41039),#68221);
#70525=DIRECTION ( 'NONE',  ( -1.000000000000000000, 0.000000000000000000, 0.000000000000000000 ) ) ;
#70677=VERTEX_POINT ( 'NONE', #21111 ) ;
#70753=DIRECTION ( 'NONE',  ( 1.000000000000000000, -0.000000000000000000, 0.000000000000000000 ) ) ;
#70784=PLANE ( 'NONE',  #27437 ) ;
#70933=ADVANCED_FACE ( 'NONE', ( #37164 ), #70784, .F. ) ;
#71024=LINE ( 'NONE', #25212, #21774 ) ;
#71053=DIRECTION ( 'NONE',  ( 0.000000000000000000, -1.000000000000000000, 8.673617379884035472E-17 ) ) ;
#71147=VERTEX_POINT ( 'NONE', #43818 ) ;
#71312=AXIS2_PLACEMENT_3D ( 'NONE', #31534, #3094, #54436 ) ;
#71319=AXIS2_PLACEMENT_3D ( 'NONE', #45144, #10069, #5621 ) ;
#71357=ORIENTED_EDGE ( 'NONE', *, *, #8966, .F. ) ;
#71366=ORIENTED_EDGE ( 'NONE', *, *, #431, .T. ) ;
#71431=DIRECTION ( 'NONE',  ( 0.000000000000000000, 1.000000000000000000, -1.040834085586083941E-14 ) ) ;
#71482=VECTOR ( 'NONE', #65866, 1000.000000000000000 ) ;
#71649=VERTEX_POINT ( 'NONE', #59513 ) ;
#71684=ADVANCED_FACE ( 'NONE', ( #59147 ), #31825, .F. ) ;
#71782=EDGE_LOOP ( 'NONE', ( #31569, #42923, #39072, #40354 ) ) ;
#71824=( NAMED_UNIT ( * ) SI_UNIT ( $, .STERADIAN. ) SOLID_ANGLE_UNIT ( ) );
#71870=DIRECTION ( 'NONE',  ( 1.000000000000000000, 0.000000000000000000, 0.000000000000000000 ) ) ;
#71888=ORIENTED_EDGE ( 'NONE', *, *, #9558, .T. ) ;
#71957=ORIENTED_EDGE ( 'NONE', *, *, #43507, .T. ) ;
#72125=ADVANCED_FACE ( 'NONE', ( #11110, #18357 ), #46, .T. ) ;
#72157=LINE ( 'NONE', #33358, #9059 ) ;
#72269=CIRCLE ( 'NONE', #69923, 9.000000000000000000 ) ;
#72302=CARTESIAN_POINT ( 'NONE',  ( 65.00000000000000000, 6.363961030679004871, 6.363961030678849440 ) ) ;
#72309=CARTESIAN_POINT ( 'NONE',  ( 65.00000000000000000, 5.218601775200109039, -7.332543590861101634 ) ) ;
#72342=DIRECTION ( 'NONE',  ( 0.000000000000000000, -8.673617379884036705E-17, -1.000000000000000000 ) ) ;
#72473=VECTOR ( 'NONE', #47949, 1000.000000000000000 ) ;
#72505=ORIENTED_EDGE ( 'NONE', *, *, #50924, .T. ) ;
#72519=CIRCLE ( 'NONE', #15868, 1.500000000000000444 ) ;
#72600=VERTEX_POINT ( 'NONE', #36823 ) ;
#72606=ORIENTED_EDGE ( 'NONE', *, *, #21587, .T. ) ;
#72711=DIRECTION ( 'NONE',  ( 0.000000000000000000, 0.000000000000000000, 1.000000000000000000 ) ) ;
#72738=ORIENTED_EDGE ( 'NONE', *, *, #1197, .F. ) ;
#72836=VECTOR ( 'NONE', #69001, 1000.000000000000000 ) ;
#72920=EDGE_LOOP ( 'NONE', ( #32950, #13381, #68447, #8572 ) ) ;
#72936=VECTOR ( 'NONE', #39699, 1000.000000000000000 ) ;
#73061=ORIENTED_EDGE ( 'NONE', *, *, #67636, .F. ) ;
#73138=COLOUR_RGB('Sky Blue',0.24,0.69,0.87);
#73139=FILL_AREA_STYLE_COLOUR('',#73138);
#73140=FILL_AREA_STYLE('',(#73139));
#73141=SURFACE_STYLE_FILL_AREA(#73140);
#73142=SURFACE_SIDE_STYLE('',(#73141));
#73143=SURFACE_STYLE_USAGE(.BOTH.,#73142);
#73144=PRESENTATION_STYLE_ASSIGNMENT((#73143));
ENDSEC;
END-ISO-10303-21;
